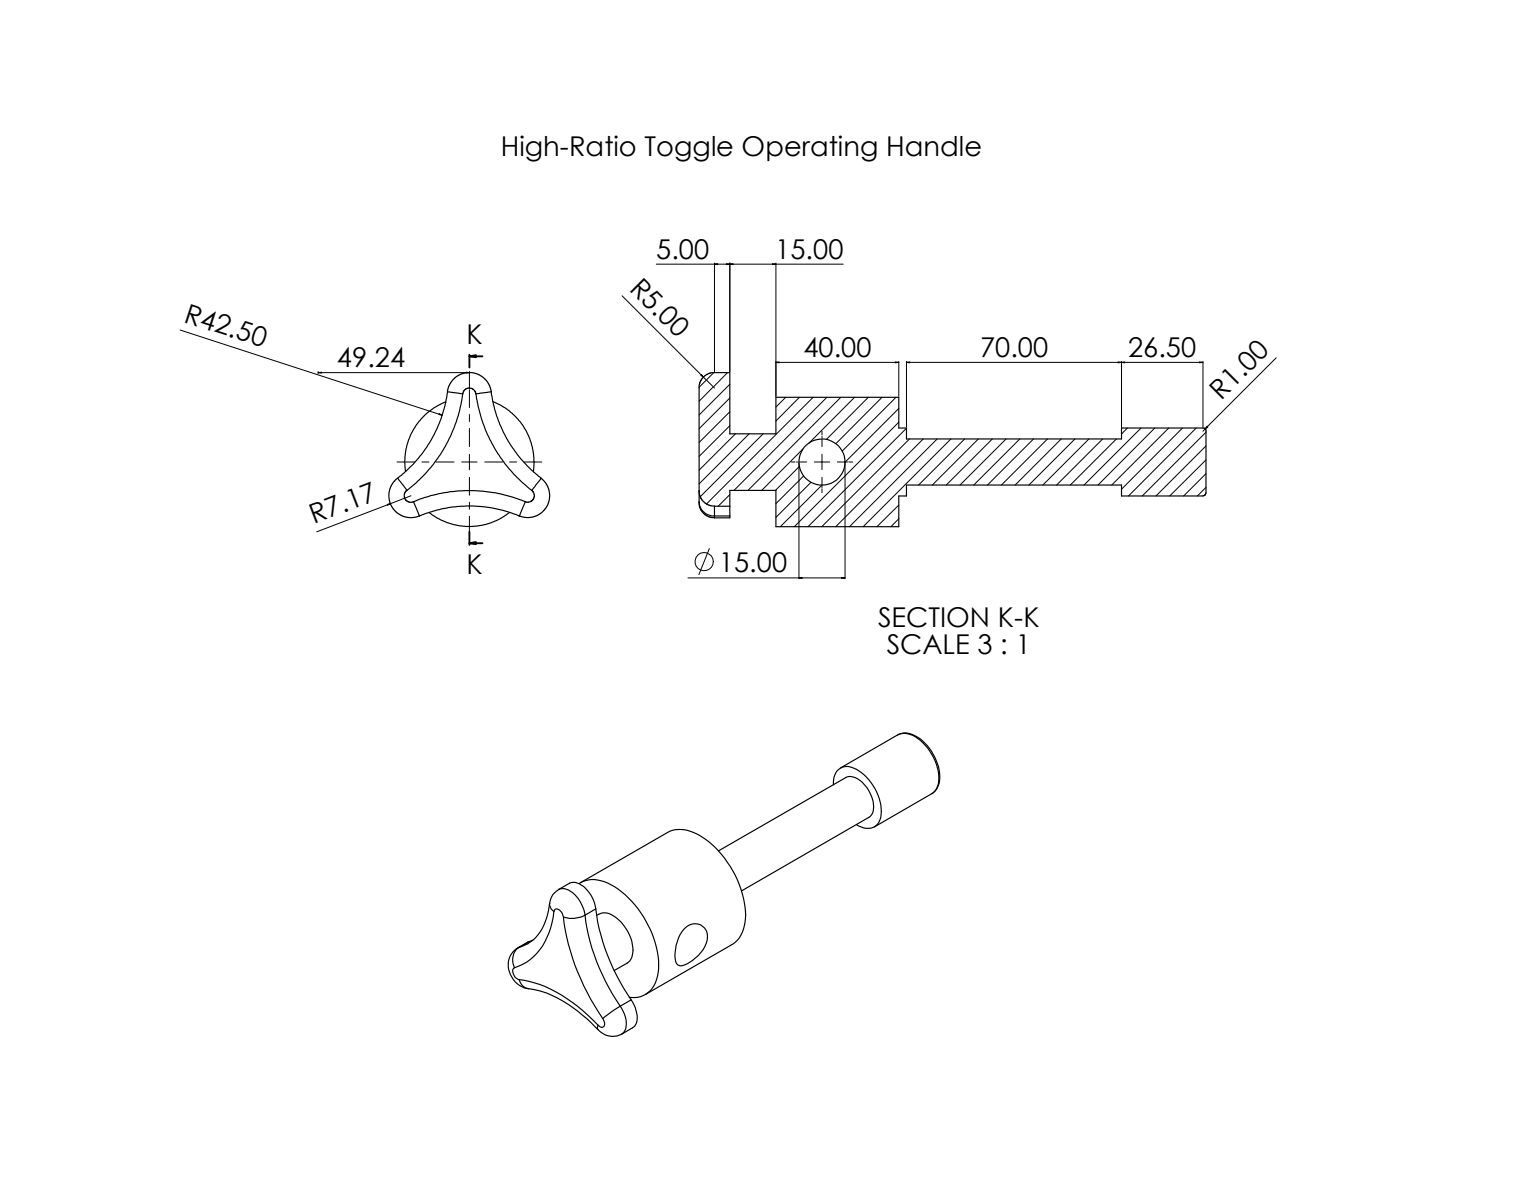
ISO-10303-21;
HEADER;
FILE_DESCRIPTION (('STEP AP214'),
    '1' );
FILE_NAME ('High-Ratio Toggle Operating Handle.step',
    '2026-10-21T18:33:49',
    ( '' ),
    ( '' ),
    'SwSTEP 2.0',
    'SolidWorks 2025',
    '' );
FILE_SCHEMA (( 'AUTOMOTIVE_DESIGN' ));
ENDSEC;

DATA;
#32=DIRECTION ( 'NONE',  ( -0.000000000000000000, -0.000000000000000000, -1.000000000000000000 ) ) ;
#36=AXIS2_PLACEMENT_3D ( 'NONE', #1369, #138, #1266 ) ;
#44=AXIS2_PLACEMENT_3D ( 'NONE', #11629, #14534, #15759 ) ;
#99=CARTESIAN_POINT ( 'NONE',  ( -57.08002265617300708, 84.22855780814606419, 35.00000000000000000 ) ) ;
#125=AXIS2_PLACEMENT_3D ( 'NONE', #2638, #18365, #4052 ) ;
#130=CYLINDRICAL_SURFACE ( 'NONE', #6082, 21.04359719766050318 ) ;
#138=DIRECTION ( 'NONE',  ( -0.000000000000000000, -0.000000000000000000, -1.000000000000000000 ) ) ;
#148=ORIENTED_EDGE ( 'NONE', *, *, #2746, .F. ) ;
#155=AXIS2_PLACEMENT_3D ( 'NONE', #551, #8645, #16166 ) ;
#219=ORIENTED_EDGE ( 'NONE', *, *, #12477, .T. ) ;
#259=CARTESIAN_POINT ( 'NONE',  ( -49.58002265617300708, 84.22855780814606419, 35.00000000000000000 ) ) ;
#264=CYLINDRICAL_SURFACE ( 'NONE', #16430, 21.04359719766050318 ) ;
#267=CARTESIAN_POINT ( 'NONE',  ( -38.92363814577095837, 71.26406042838981136, 102.5000000000000000 ) ) ;
#313=ORIENTED_EDGE ( 'NONE', *, *, #10756, .F. ) ;
#314=MANIFOLD_SOLID_BREP ( 'Cut-Extrude8', #12995 ) ;
#315=VERTEX_POINT ( 'NONE', #4152 ) ;
#323=DIRECTION ( 'NONE',  ( 0.000000000000000000, 0.000000000000000000, -1.000000000000000000 ) ) ;
#335=EDGE_CURVE ( 'NONE', #5779, #10128, #2839, .T. ) ;
#350=CARTESIAN_POINT ( 'NONE',  ( -83.23321842955245131, 73.26749283226919829, 97.49999999999998579 ) ) ;
#356=LINE ( 'NONE', #17469, #14795 ) ;
#358=CARTESIAN_POINT ( 'NONE',  ( -37.24050225201523290, 91.24541864506342392, 59.84040329251897816 ) ) ;
#361=ADVANCED_FACE ( 'NONE', ( #3024 ), #9005, .T. ) ;
#365=VECTOR ( 'NONE', #12626, 1000.000000000000000 ) ;
#377=CARTESIAN_POINT ( 'NONE',  ( -77.86181869377003295, 80.88798785482902076, 69.23289521281527925 ) ) ;
#408=LINE ( 'NONE', #4696, #15529 ) ;
#421=DIRECTION ( 'NONE',  ( -1.000000000000000000, 0.000000000000000000, 0.000000000000000000 ) ) ;
#449=CIRCLE ( 'NONE', #2236, 21.04359719766049608 ) ;
#456=DIRECTION ( 'NONE',  ( 0.000000000000000000, 0.000000000000000000, 1.000000000000000000 ) ) ;
#461=CARTESIAN_POINT ( 'NONE',  ( -36.29822661857599542, 80.88798785482900655, 55.76710478718474917 ) ) ;
#470=CARTESIAN_POINT ( 'NONE',  ( -73.32517902883354566, 66.64375664990241432, 102.5000000000000000 ) ) ;
#512=DIRECTION ( 'NONE',  ( 0.000000000000000000, 0.000000000000000000, 1.000000000000000000 ) ) ;
#534=CARTESIAN_POINT ( 'NONE',  ( -36.04074381574865527, 84.72093613475881568, 69.98790959730909833 ) ) ;
#551=CARTESIAN_POINT ( 'NONE',  ( -57.08002265617301418, 106.1506877598988154, 97.49999999999998579 ) ) ;
#554=ORIENTED_EDGE ( 'NONE', *, *, #15682, .F. ) ;
#569=TOROIDAL_SURFACE ( 'NONE', #11925, 10.04359719766049963, 1.000000000000000000 ) ;
#592=CIRCLE ( 'NONE', #14907, 7.168074330098680669 ) ;
#595=CARTESIAN_POINT ( 'NONE',  ( -78.12361985383350316, 84.22855780814606419, 77.50000000000000000 ) ) ;
#598=DIRECTION ( 'NONE',  ( 0.000000000000000000, 0.000000000000000000, 1.000000000000000000 ) ) ;
#604=AXIS2_PLACEMENT_3D ( 'NONE', #7949, #3633, #837 ) ;
#610=B_SPLINE_CURVE_WITH_KNOTS ( 'NONE', 3,
 ( #15647, #8545, #1426, #14249, #5805, #17565, #12326, #377, #10719, #3183, #10817, #4747, #15119, #3714, #16415, #3604, #897, #9324, #15203, #10926, #9506, #8984, #5202, #15020, #6601, #11795, #10297, #18019, #2389, #3804, #8096, #8894, #16611, #14677, #12219, #2299, #13815, #1004, #2211, #8002, #12429, #6705, #16072, #13198, #6066, #16515 ),
 .UNSPECIFIED., .F., .F.,
 ( 4, 2, 2, 2, 2, 2, 2, 2, 2, 2, 2, 2, 2, 2, 2, 2, 2, 2, 2, 2, 2, 2, 4 ),
 ( 1.387778780781445676E-17, 0.001477780233738794748, 0.002216670350608189195, 0.002955560467477583424, 0.004433340701216313337, 0.005172230818085679811, 0.005911120934955047153, 0.007388901168693846888, 0.008866681402432645756, 0.009605571519302056466, 0.01034446163617146891, 0.01182224186991029206, 0.01330002210364911869, 0.01477780233738794531, 0.01625558257112677193, 0.01699447268799620173, 0.01773336280486562805, 0.01921114303860447722, 0.01995003315547392089, 0.02068892327234336456, 0.02216670350608221027, 0.02290559362295161577, 0.02364448373982101781 ),
 .UNSPECIFIED. ) ;
#627=CIRCLE ( 'NONE', #12604, 47.49926016644946714 ) ;
#634=AXIS2_PLACEMENT_3D ( 'NONE', #7986, #512, #13420 ) ;
#641=EDGE_LOOP ( 'NONE', ( #13099, #15798 ) ) ;
#647=AXIS2_PLACEMENT_3D ( 'NONE', #8443, #1344, #3846 ) ;
#674=CARTESIAN_POINT ( 'NONE',  ( -76.06514409945376087, 73.26749283226919829, 97.49999999999998579 ) ) ;
#715=VERTEX_POINT ( 'NONE', #12761 ) ;
#718=DIRECTION ( 'NONE',  ( -1.000000000000000000, 0.000000000000000000, 0.000000000000000000 ) ) ;
#742=CARTESIAN_POINT ( 'NONE',  ( -36.67168494155210112, 79.09395985567564935, 57.02782509738743499 ) ) ;
#779=CARTESIAN_POINT ( 'NONE',  ( -76.88569266382195622, 91.34252568597634081, 60.07430202819471532 ) ) ;
#803=EDGE_CURVE ( 'NONE', #10920, #7762, #4578, .T. ) ;
#837=DIRECTION ( 'NONE',  ( 1.000000000000000000, 0.000000000000000000, 0.000000000000000000 ) ) ;
#851=UNCERTAINTY_MEASURE_WITH_UNIT (LENGTH_MEASURE( 1.000000000000000082E-05 ), #7064, 'distance_accuracy_value', 'NONE');
#856=CARTESIAN_POINT ( 'NONE',  ( -68.12361985383350316, 84.22855780814606419, 68.73600986863397111 ) ) ;
#861=CARTESIAN_POINT ( 'NONE',  ( -78.11930149659737310, 84.72093613475881568, 55.01209040269093720 ) ) ;
#868=FACE_OUTER_BOUND ( 'NONE', #12414, .T. ) ;
#872=EDGE_LOOP ( 'NONE', ( #7610, #14353 ) ) ;
#874=CARTESIAN_POINT ( 'NONE',  ( -38.92363814577095837, 71.26406042838981136, 97.49999999999998579 ) ) ;
#896=DIRECTION ( 'NONE',  ( -1.000000000000000000, 0.000000000000000000, 0.000000000000000000 ) ) ;
#897=CARTESIAN_POINT ( 'NONE',  ( -77.01756027604902499, 77.49305091727374872, 65.83480828159299847 ) ) ;
#918=ADVANCED_FACE ( 'NONE', ( #16269 ), #6147, .T. ) ;
#964=CARTESIAN_POINT ( 'NONE',  ( -77.95646096175848072, 86.88560906486408442, 69.51788182020753482 ) ) ;
#970=ORIENTED_EDGE ( 'NONE', *, *, #15172, .F. ) ;
#981=ORIENTED_EDGE ( 'NONE', *, *, #2192, .T. ) ;
#1004=CARTESIAN_POINT ( 'NONE',  ( -77.85981289659012816, 80.89962780276930232, 55.77475785633962602 ) ) ;
#1052=EDGE_CURVE ( 'NONE', #6388, #2078, #4951, .T. ) ;
#1066=ORIENTED_EDGE ( 'NONE', *, *, #5722, .T. ) ;
#1070=CARTESIAN_POINT ( 'NONE',  ( -77.35494310313409017, 89.87539756129700663, 67.45979609325928550 ) ) ;
#1071=EDGE_LOOP ( 'NONE', ( #14079, #1438 ) ) ;
#1095=ORIENTED_EDGE ( 'NONE', *, *, #8907, .T. ) ;
#1097=CYLINDRICAL_SURFACE ( 'NONE', #4269, 7.168074330098680669 ) ;
#1137=ORIENTED_EDGE ( 'NONE', *, *, #12714, .F. ) ;
#1180=DIRECTION ( 'NONE',  ( -1.000000000000000000, 0.000000000000000000, 0.000000000000000000 ) ) ;
#1186=ADVANCED_FACE ( 'NONE', ( #7022 ), #9528, .F. ) ;
#1207=CARTESIAN_POINT ( 'NONE',  ( -68.12361985383350316, 84.22855780814606419, 37.50000000000000000 ) ) ;
#1224=AXIS2_PLACEMENT_3D ( 'NONE', #99, #12928, #17214 ) ;
#1228=LINE ( 'NONE', #4398, #12878 ) ;
#1238=DIRECTION ( 'NONE',  ( 0.000000000000000000, 0.000000000000000000, 1.000000000000000000 ) ) ;
#1241=CARTESIAN_POINT ( 'NONE',  ( -83.23321842955245131, 73.26749283226919829, 92.50000000000000000 ) ) ;
#1252=CARTESIAN_POINT ( 'NONE',  ( -38.09490121289055509, 73.26749283227019305, 97.49999999999998579 ) ) ;
#1266=DIRECTION ( 'NONE',  ( -1.000000000000000000, 0.000000000000000000, 0.000000000000000000 ) ) ;
#1341=DIRECTION ( 'NONE',  ( -1.000000000000000000, 0.000000000000000000, 0.000000000000000000 ) ) ;
#1344=DIRECTION ( 'NONE',  ( -0.000000000000000000, 0.000000000000000000, -1.000000000000000000 ) ) ;
#1354=CARTESIAN_POINT ( 'NONE',  ( -76.06514409945376087, 73.26749283226919829, 102.5000000000000000 ) ) ;
#1355=VECTOR ( 'NONE', #4745, 1000.000000000000000 ) ;
#1369=CARTESIAN_POINT ( 'NONE',  ( -106.3193689061042164, 112.6569076202650450, 97.49999999999998579 ) ) ;
#1380=ORIENTED_EDGE ( 'NONE', *, *, #3456, .T. ) ;
#1395=DIRECTION ( 'NONE',  ( -0.000000000000000000, -0.000000000000000000, -1.000000000000000000 ) ) ;
#1420=EDGE_LOOP ( 'NONE', ( #3178, #16210, #16979, #14921 ) ) ;
#1426=CARTESIAN_POINT ( 'NONE',  ( -78.10583824988592028, 83.23774243329727085, 69.95051152545947559 ) ) ;
#1438=ORIENTED_EDGE ( 'NONE', *, *, #14205, .T. ) ;
#1441=CARTESIAN_POINT ( 'NONE',  ( -57.08002265617300708, 84.22855780814606419, 77.50000000000000000 ) ) ;
#1495=CARTESIAN_POINT ( 'NONE',  ( -57.08002265617300708, 84.22855780814606419, 92.50000000000000000 ) ) ;
#1508=CARTESIAN_POINT ( 'NONE',  ( -80.43148536604020649, 78.95224028009165806, 102.5000000000000000 ) ) ;
#1537=ORIENTED_EDGE ( 'NONE', *, *, #14930, .T. ) ;
#1540=DIRECTION ( 'NONE',  ( -1.000000000000000000, 0.000000000000000000, 0.000000000000000000 ) ) ;
#1583=CARTESIAN_POINT ( 'NONE',  ( -36.05803997522690452, 85.21341043856776309, 69.93917279341883386 ) ) ;
#1589=CYLINDRICAL_SURFACE ( 'NONE', #16728, 7.168074330099291736 ) ;
#1663=FACE_OUTER_BOUND ( 'NONE', #16501, .T. ) ;
#1672=DIRECTION ( 'NONE',  ( -1.000000000000000000, 0.000000000000000000, 0.000000000000000000 ) ) ;
#1676=CARTESIAN_POINT ( 'NONE',  ( -37.41836177203395408, 91.72869609463791107, 62.99211610237011172 ) ) ;
#1689=EDGE_CURVE ( 'NONE', #11390, #9243, #16057, .T. ) ;
#1711=PLANE ( 'NONE',  #44 ) ;
#1729=CARTESIAN_POINT ( 'NONE',  ( -76.06514409945376087, 73.26749283226919829, 92.50000000000000000 ) ) ;
#1735=CYLINDRICAL_SURFACE ( 'NONE', #9620, 9.197489084949710403 ) ;
#1758=CARTESIAN_POINT ( 'NONE',  ( -36.37230694946377696, 87.99602245404176415, 55.99668402450813431 ) ) ;
#1788=ORIENTED_EDGE ( 'NONE', *, *, #335, .F. ) ;
#1796=DIRECTION ( 'NONE',  ( 0.3822456275482439270, -0.9240607556975077852, 0.000000000000000000 ) ) ;
#1801=LINE ( 'NONE', #8920, #18007 ) ;
#1853=DIRECTION ( 'NONE',  ( -0.000000000000000000, -0.000000000000000000, -1.000000000000000000 ) ) ;
#1862=CARTESIAN_POINT ( 'NONE',  ( -36.12589806422543148, 82.27553650601718971, 55.25452123045118213 ) ) ;
#1872=CIRCLE ( 'NONE', #13239, 9.197489084949710403 ) ;
#1953=DIRECTION ( 'NONE',  ( 1.000000000000000000, 0.000000000000000000, -0.000000000000000000 ) ) ;
#1970=DIRECTION ( 'NONE',  ( 1.000000000000000000, 0.000000000000000000, 0.000000000000000000 ) ) ;
#1978=B_SPLINE_CURVE_WITH_KNOTS ( 'NONE', 3,
 ( #4661, #10374, #3254, #14669, #1862, #7570, #13280, #461, #10834, #4010, #15036, #9438, #742, #17932, #9522, #17844, #6619, #11027, #6520, #2229, #3622, #15132, #2314, #16531, #9723, #7941, #8020, #6435, #5117, #15224, #5021, #12343, #16712, #12236, #9616, #2410, #2612, #10940, #13733, #15320, #12533, #13651, #8116, #6724, #13554, #6812 ),
 .UNSPECIFIED., .F., .F.,
 ( 4, 2, 2, 2, 2, 2, 2, 2, 2, 2, 2, 2, 2, 2, 2, 2, 2, 2, 2, 2, 2, 2, 4 ),
 ( 0.000000000000000000, 0.001477780233738735334, 0.002216670350608105061, 0.002955560467477474570, 0.004433340701216251754, 0.005172230818085658995, 0.005911120934955066235, 0.007388901168693925818, 0.008866681402432782799, 0.009605571519302205652, 0.01034446163617162677, 0.01182224186991048982, 0.01330002210364935461, 0.01477780233738821593, 0.01625558257112707725, 0.01699447268799647928, 0.01773336280486588479, 0.01921114303860466457, 0.01995003315547405273, 0.02068892327234343395, 0.02216670350608219292, 0.02290559362295159149, 0.02364448373982099005 ),
 .UNSPECIFIED. ) ;
#1991=CARTESIAN_POINT ( 'NONE',  ( -76.83309350041878361, 91.48526692943183036, 60.54251226750088222 ) ) ;
#1994=DIRECTION ( 'NONE',  ( -1.000000000000000000, 0.000000000000000000, 0.000000000000000000 ) ) ;
#2010=EDGE_CURVE ( 'NONE', #8653, #11390, #6438, .T. ) ;
#2014=ORIENTED_EDGE ( 'NONE', *, *, #2838, .F. ) ;
#2026=CARTESIAN_POINT ( 'NONE',  ( -47.88253357122329845, 84.22855780814606419, 92.50000000000000000 ) ) ;
#2064=EDGE_CURVE ( 'NONE', #14012, #2549, #12075, .T. ) ;
#2078=VERTEX_POINT ( 'NONE', #3533 ) ;
#2092=ORIENTED_EDGE ( 'NONE', *, *, #4008, .T. ) ;
#2169=CARTESIAN_POINT ( 'NONE',  ( -78.23321842955243710, 73.26749283226919829, 97.49999999999998579 ) ) ;
#2173=FACE_OUTER_BOUND ( 'NONE', #18405, .T. ) ;
#2181=AXIS2_PLACEMENT_3D ( 'NONE', #6034, #4384, #2976 ) ;
#2192=EDGE_CURVE ( 'NONE', #8653, #10149, #14444, .T. ) ;
#2194=( GEOMETRIC_REPRESENTATION_CONTEXT ( 3 ) GLOBAL_UNCERTAINTY_ASSIGNED_CONTEXT ( ( #12468 ) ) GLOBAL_UNIT_ASSIGNED_CONTEXT ( ( #10446, #10543, #16139 ) ) REPRESENTATION_CONTEXT ( 'NONE', 'WORKASPACE' ) );
#2195=AXIS2_PLACEMENT_3D ( 'NONE', #3510, #5002, #17909 ) ;
#2211=CARTESIAN_POINT ( 'NONE',  ( -77.89415131665849401, 81.12099773066752562, 55.66971324650689468 ) ) ;
#2227=PRODUCT_DEFINITION ( 'UNKNOWN', '', #11173, #6257 ) ;
#2229=CARTESIAN_POINT ( 'NONE',  ( -37.32251811057857793, 76.98425793134822470, 60.54272255928178481 ) ) ;
#2236=AXIS2_PLACEMENT_3D ( 'NONE', #5521, #18049, #2427 ) ;
#2248=EDGE_CURVE ( 'NONE', #4300, #12168, #2317, .T. ) ;
#2259=DIRECTION ( 'NONE',  ( -0.000000000000000000, -0.000000000000000000, -1.000000000000000000 ) ) ;
#2299=CARTESIAN_POINT ( 'NONE',  ( -77.74594894602464024, 80.25424057604627137, 56.13491590375404172 ) ) ;
#2314=CARTESIAN_POINT ( 'NONE',  ( -37.41820911104731806, 76.72881973191589111, 62.00219528655608059 ) ) ;
#2317=LINE ( 'NONE', #8024, #6348 ) ;
#2340=DIRECTION ( 'NONE',  ( -0.000000000000000000, -0.000000000000000000, -1.000000000000000000 ) ) ;
#2343=CARTESIAN_POINT ( 'NONE',  ( -40.83486628351231218, 66.64375664990294013, 97.49999999999998579 ) ) ;
#2389=CARTESIAN_POINT ( 'NONE',  ( -77.09623126797262671, 77.72742355542474968, 58.72881290435446289 ) ) ;
#2400=ADVANCED_FACE ( 'NONE', ( #1663 ), #16049, .T. ) ;
#2408=CARTESIAN_POINT ( 'NONE',  ( -57.08002265617300708, 84.22855780814606419, 68.73600986863397111 ) ) ;
#2410=CARTESIAN_POINT ( 'NONE',  ( -36.41409636632135971, 80.25424057604624295, 68.86508409624599381 ) ) ;
#2414=EDGE_CURVE ( 'NONE', #10920, #17012, #10253, .T. ) ;
#2421=EDGE_CURVE ( 'NONE', #17891, #4300, #13836, .T. ) ;
#2427=DIRECTION ( 'NONE',  ( 1.000000000000000000, 0.000000000000000000, 0.000000000000000000 ) ) ;
#2453=CARTESIAN_POINT ( 'NONE',  ( -76.76049879875490944, 91.67990741037235125, 63.48630363751230021 ) ) ;
#2462=AXIS2_PLACEMENT_3D ( 'NONE', #6172, #2259, #13314 ) ;
#2467=DIRECTION ( 'NONE',  ( -0.000000000000000000, -0.000000000000000000, 1.000000000000000000 ) ) ;
#2484=CARTESIAN_POINT ( 'NONE',  ( -7.840676406241780860, 112.6569076202650308, 92.50000000000000000 ) ) ;
#2499=ORIENTED_EDGE ( 'NONE', *, *, #12714, .T. ) ;
#2514=ORIENTED_EDGE ( 'NONE', *, *, #3214, .T. ) ;
#2549=VERTEX_POINT ( 'NONE', #16234 ) ;
#2563=CARTESIAN_POINT ( 'NONE',  ( -78.12361985383350316, 84.22855780814607840, 70.00000000000001421 ) ) ;
#2586=CARTESIAN_POINT ( 'NONE',  ( -57.08002265617300708, 84.22855780814606419, 35.00000000000000000 ) ) ;
#2589=CARTESIAN_POINT ( 'NONE',  ( -54.93063083320800644, 106.4346967249107792, 97.49999999999998579 ) ) ;
#2594=DIRECTION ( 'NONE',  ( -1.224646799147353207E-16, 1.000000000000000000, 0.000000000000000000 ) ) ;
#2597=DIRECTION ( 'NONE',  ( -0.000000000000000000, -0.000000000000000000, -1.000000000000000000 ) ) ;
#2612=CARTESIAN_POINT ( 'NONE',  ( -36.37443156682203949, 80.46558623543624833, 68.99235718476280965 ) ) ;
#2622=DIRECTION ( 'NONE',  ( -1.000000000000000000, 0.000000000000000000, 0.000000000000000000 ) ) ;
#2627=ORIENTED_EDGE ( 'NONE', *, *, #12477, .F. ) ;
#2638=CARTESIAN_POINT ( 'NONE',  ( -38.09490121289055509, 73.26749283227019305, 97.49999999999998579 ) ) ;
#2653=FACE_OUTER_BOUND ( 'NONE', #13653, .T. ) ;
#2657=EDGE_CURVE ( 'NONE', #17012, #4505, #3991, .T. ) ;
#2670=ORIENTED_EDGE ( 'NONE', *, *, #14218, .T. ) ;
#2671=PLANE ( 'NONE',  #15226 ) ;
#2687=CARTESIAN_POINT ( 'NONE',  ( -57.08002265617300708, 84.22855780814606419, -35.00000000000000000 ) ) ;
#2693=LINE ( 'NONE', #6714, #365 ) ;
#2746=EDGE_CURVE ( 'NONE', #5564, #15197, #8172, .T. ) ;
#2747=EDGE_LOOP ( 'NONE', ( #8359, #11367 ) ) ;
#2749=DIRECTION ( 'NONE',  ( 0.000000000000000000, 0.000000000000000000, -1.000000000000000000 ) ) ;
#2778=EDGE_CURVE ( 'NONE', #15227, #15032, #7428, .T. ) ;
#2786=VERTEX_POINT ( 'NONE', #595 ) ;
#2838=EDGE_CURVE ( 'NONE', #9739, #15151, #17147, .T. ) ;
#2839=CIRCLE ( 'NONE', #13284, 10.04359719766049430 ) ;
#2890=DIRECTION ( 'NONE',  ( -1.000000000000000000, 0.000000000000000000, 0.000000000000000000 ) ) ;
#2893=ADVANCED_FACE ( 'NONE', ( #5274 ), #16765, .T. ) ;
#2911=EDGE_CURVE ( 'NONE', #15151, #8454, #17991, .T. ) ;
#2935=FACE_OUTER_BOUND ( 'NONE', #17821, .T. ) ;
#2938=ADVANCED_FACE ( 'NONE', ( #2935 ), #130, .T. ) ;
#2944=DIRECTION ( 'NONE',  ( -1.000000000000000000, 0.000000000000000000, 0.000000000000000000 ) ) ;
#2963=CARTESIAN_POINT ( 'NONE',  ( -64.18632899337946185, 107.0896764944433954, 102.5000000000000000 ) ) ;
#2976=DIRECTION ( 'NONE',  ( -1.000000000000000000, -1.632709340522812220E-15, 0.000000000000000000 ) ) ;
#2990=CARTESIAN_POINT ( 'NONE',  ( -37.13913369598539305, 90.95230598576922887, 65.83182832201505619 ) ) ;
#2991=DIRECTION ( 'NONE',  ( 1.000000000000000000, 0.000000000000000000, 0.000000000000000000 ) ) ;
#3013=ORIENTED_EDGE ( 'NONE', *, *, #17161, .T. ) ;
#3024=FACE_OUTER_BOUND ( 'NONE', #1420, .T. ) ;
#3030=FACE_OUTER_BOUND ( 'NONE', #3216, .T. ) ;
#3040=ORIENTED_EDGE ( 'NONE', *, *, #15682, .T. ) ;
#3059=CARTESIAN_POINT ( 'NONE',  ( -78.12361985383350316, 84.22855780814606419, 37.50000000000000000 ) ) ;
#3077=CARTESIAN_POINT ( 'NONE',  ( -37.02218768164058815, 90.59536451873519525, 66.47148242010926822 ) ) ;
#3095=DIRECTION ( 'NONE',  ( -1.000000000000000000, 0.000000000000000000, 0.000000000000000000 ) ) ;
#3136=CARTESIAN_POINT ( 'NONE',  ( -57.08002265617300708, 84.22855780814606419, 37.50000000000000000 ) ) ;
#3155=CIRCLE ( 'NONE', #8835, 42.49926016644912607 ) ;
#3165=CARTESIAN_POINT ( 'NONE',  ( -66.27751174112272281, 84.22855780814606419, 77.50000000000000000 ) ) ;
#3172=CARTESIAN_POINT ( 'NONE',  ( -37.06251219239532446, 90.72064142110004070, 58.73664414705599768 ) ) ;
#3173=PLANE ( 'NONE',  #17051 ) ;
#3178=ORIENTED_EDGE ( 'NONE', *, *, #4773, .F. ) ;
#3183=CARTESIAN_POINT ( 'NONE',  ( -77.66397652102858729, 79.84943054288078201, 68.59368636907963435 ) ) ;
#3194=DIRECTION ( 'NONE',  ( 1.000000000000000000, 0.000000000000000000, 0.000000000000000000 ) ) ;
#3214=EDGE_CURVE ( 'NONE', #15197, #15151, #12698, .T. ) ;
#3216=EDGE_LOOP ( 'NONE', ( #8491, #17094, #10489, #14441 ) ) ;
#3239=DIRECTION ( 'NONE',  ( -1.000000000000000000, 0.000000000000000000, -0.000000000000000000 ) ) ;
#3243=AXIS2_PLACEMENT_3D ( 'NONE', #10958, #9363, #16732 ) ;
#3254=CARTESIAN_POINT ( 'NONE',  ( -36.05420706246012230, 83.23774243329727085, 55.04948847454055283 ) ) ;
#3281=CIRCLE ( 'NONE', #7774, 7.168074330098680669 ) ;
#3310=EDGE_CURVE ( 'NONE', #15460, #7762, #15952, .T. ) ;
#3336=CARTESIAN_POINT ( 'NONE',  ( -83.23321842955245131, 73.26749283226919829, 102.5000000000000000 ) ) ;
#3339=CARTESIAN_POINT ( 'NONE',  ( -36.29790135706344500, 87.56725157785861313, 55.76609545620163999 ) ) ;
#3366=EDGE_LOOP ( 'NONE', ( #8412, #7266 ) ) ;
#3373=AXIS2_PLACEMENT_3D ( 'NONE', #5947, #13260, #14388 ) ;
#3383=CARTESIAN_POINT ( 'NONE',  ( -77.02091161636059269, 90.95230598576924308, 59.16817167798495802 ) ) ;
#3410=EDGE_CURVE ( 'NONE', #15435, #4264, #6845, .T. ) ;
#3431=AXIS2_PLACEMENT_3D ( 'NONE', #2589, #9692, #6880 ) ;
#3448=EDGE_LOOP ( 'NONE', ( #17964, #7792, #4837, #16368, #8677, #11944, #5495 ) ) ;
#3456=EDGE_CURVE ( 'NONE', #2549, #14012, #610, .T. ) ;
#3463=DIRECTION ( 'NONE',  ( 0.000000000000000000, 0.000000000000000000, 1.000000000000000000 ) ) ;
#3480=DIRECTION ( 'NONE',  ( 0.000000000000000000, 0.000000000000000000, -1.000000000000000000 ) ) ;
#3497=CARTESIAN_POINT ( 'NONE',  ( -36.03642545851251100, 84.22855780814606419, 37.50000000000000000 ) ) ;
#3505=DIRECTION ( 'NONE',  ( -1.000000000000000000, 0.000000000000000000, 0.000000000000000000 ) ) ;
#3510=CARTESIAN_POINT ( 'NONE',  ( -57.08002265617300708, 84.22855780814606419, 77.50000000000000000 ) ) ;
#3533=CARTESIAN_POINT ( 'NONE',  ( -73.32517902883354566, 66.64375664990241432, 92.50000000000000000 ) ) ;
#3563=DIRECTION ( 'NONE',  ( -0.000000000000000000, -0.000000000000000000, -1.000000000000000000 ) ) ;
#3564=AXIS2_PLACEMENT_3D ( 'NONE', #674, #3563, #6757 ) ;
#3569=CARTESIAN_POINT ( 'NONE',  ( -77.62243764337172536, 88.81248391902214223, 56.54393065445481881 ) ) ;
#3571=ORIENTED_EDGE ( 'NONE', *, *, #4773, .T. ) ;
#3572=FACE_OUTER_BOUND ( 'NONE', #9361, .T. ) ;
#3577=AXIS2_PLACEMENT_3D ( 'NONE', #13659, #12355, #4954 ) ;
#3604=CARTESIAN_POINT ( 'NONE',  ( -77.09486422618832080, 77.72307496574235586, 66.26442681581322347 ) ) ;
#3614=ORIENTED_EDGE ( 'NONE', *, *, #14205, .F. ) ;
#3622=CARTESIAN_POINT ( 'NONE',  ( -37.34515446474368616, 76.92303621577349304, 60.78520344204553538 ) ) ;
#3623=ORIENTED_EDGE ( 'NONE', *, *, #2064, .F. ) ;
#3633=DIRECTION ( 'NONE',  ( -0.000000000000000000, -0.000000000000000000, -1.000000000000000000 ) ) ;
#3677=FACE_OUTER_BOUND ( 'NONE', #6379, .T. ) ;
#3682=AXIS2_PLACEMENT_3D ( 'NONE', #17936, #9442, #16535 ) ;
#3712=CARTESIAN_POINT ( 'NONE',  ( -36.03642545851251100, 84.22855780814606419, 77.50000000000000000 ) ) ;
#3714=CARTESIAN_POINT ( 'NONE',  ( -77.35440395286859427, 78.57985073358727846, 67.45754834358830010 ) ) ;
#3724=AXIS2_PLACEMENT_3D ( 'NONE', #2687, #9894, #8499 ) ;
#3735=AXIS2_PLACEMENT_3D ( 'NONE', #13528, #5193, #3505 ) ;
#3746=ORIENTED_EDGE ( 'NONE', *, *, #2192, .F. ) ;
#3750=DIRECTION ( 'NONE',  ( -0.000000000000000000, -0.000000000000000000, -1.000000000000000000 ) ) ;
#3752=ORIENTED_EDGE ( 'NONE', *, *, #8089, .F. ) ;
#3759=ADVANCED_FACE ( 'NONE', ( #10246 ), #14466, .T. ) ;
#3760=LINE ( 'NONE', #856, #8958 ) ;
#3765=VERTEX_POINT ( 'NONE', #14629 ) ;
#3780=EDGE_CURVE ( 'NONE', #4264, #10128, #7159, .T. ) ;
#3800=DIRECTION ( 'NONE',  ( -0.000000000000000000, -0.000000000000000000, -1.000000000000000000 ) ) ;
#3804=CARTESIAN_POINT ( 'NONE',  ( -77.22213323485729575, 78.13360439242252653, 58.12270716872546927 ) ) ;
#3819=ORIENTED_EDGE ( 'NONE', *, *, #14218, .F. ) ;
#3846=DIRECTION ( 'NONE',  ( -1.000000000000000000, 0.000000000000000000, 0.000000000000000000 ) ) ;
#3883=ORIENTED_EDGE ( 'NONE', *, *, #5854, .F. ) ;
#3885=CARTESIAN_POINT ( 'NONE',  ( -35.92682688279126779, 73.26749283227019305, 97.49999999999998579 ) ) ;
#3893=ADVANCED_FACE ( 'NONE', ( #18398, #15289 ), #2671, .F. ) ;
#3915=AXIS2_PLACEMENT_3D ( 'NONE', #14702, #7413, #1796 ) ;
#3921=AXIS2_PLACEMENT_3D ( 'NONE', #16023, #10138, #2944 ) ;
#3924=ORIENTED_EDGE ( 'NONE', *, *, #16449, .T. ) ;
#3943=FACE_OUTER_BOUND ( 'NONE', #3448, .T. ) ;
#3946=DIRECTION ( 'NONE',  ( 1.000000000000000000, 0.000000000000000000, 0.000000000000000000 ) ) ;
#3948=CARTESIAN_POINT ( 'NONE',  ( -77.53399986885767703, 89.18779308299872355, 68.14733228818110433 ) ) ;
#3957=ORIENTED_EDGE ( 'NONE', *, *, #4008, .F. ) ;
#3959=AXIS2_PLACEMENT_3D ( 'NONE', #14352, #7416, #1540 ) ;
#3973=CARTESIAN_POINT ( 'NONE',  ( -38.09490121289055509, 73.26749283227019305, 102.5000000000000000 ) ) ;
#3980=ORIENTED_EDGE ( 'NONE', *, *, #5034, .T. ) ;
#3991=CIRCLE ( 'NONE', #10264, 4.999999999999998224 ) ;
#4008=EDGE_CURVE ( 'NONE', #8703, #8868, #4519, .T. ) ;
#4010=CARTESIAN_POINT ( 'NONE',  ( -36.49606879131744108, 79.84943054288081044, 56.40631363092040829 ) ) ;
#4011=ORIENTED_EDGE ( 'NONE', *, *, #2838, .T. ) ;
#4036=ORIENTED_EDGE ( 'NONE', *, *, #1052, .T. ) ;
#4038=EDGE_CURVE ( 'NONE', #715, #6290, #9548, .T. ) ;
#4045=AXIS2_PLACEMENT_3D ( 'NONE', #5357, #8370, #11465 ) ;
#4052=DIRECTION ( 'NONE',  ( -1.000000000000000000, 0.000000000000000000, 0.000000000000000000 ) ) ;
#4082=CARTESIAN_POINT ( 'NONE',  ( -76.06514409945376087, 73.26749283226919829, 102.5000000000000000 ) ) ;
#4089=ORIENTED_EDGE ( 'NONE', *, *, #4353, .T. ) ;
#4130=ADVANCED_FACE ( 'NONE', ( #2173 ), #569, .T. ) ;
#4147=VERTEX_POINT ( 'NONE', #10690 ) ;
#4148=DIRECTION ( 'NONE',  ( -1.000000000000000000, 0.000000000000000000, 0.000000000000000000 ) ) ;
#4150=ADVANCED_FACE ( 'NONE', ( #3572 ), #9113, .T. ) ;
#4152=CARTESIAN_POINT ( 'NONE',  ( -64.58002265617299997, 84.22855780814606419, -35.00000000000000000 ) ) ;
#4153=CIRCLE ( 'NONE', #6834, 11.04359719766050141 ) ;
#4167=ORIENTED_EDGE ( 'NONE', *, *, #2778, .F. ) ;
#4239=EDGE_CURVE ( 'NONE', #2549, #7660, #408, .T. ) ;
#4264=VERTEX_POINT ( 'NONE', #15167 ) ;
#4269=AXIS2_PLACEMENT_3D ( 'NONE', #4082, #12700, #18399 ) ;
#4292=CYLINDRICAL_SURFACE ( 'NONE', #15254, 42.49926016645017057 ) ;
#4299=CARTESIAN_POINT ( 'NONE',  ( -68.12361985383350316, 84.22855780814606419, -35.00000000000000000 ) ) ;
#4300=VERTEX_POINT ( 'NONE', #5167 ) ;
#4332=CYLINDRICAL_SURFACE ( 'NONE', #15784, 7.168074330098680669 ) ;
#4353=EDGE_CURVE ( 'NONE', #14012, #8703, #6952, .T. ) ;
#4356=TOROIDAL_SURFACE ( 'NONE', #10326, 2.168074330098679336, 5.000000000000000000 ) ;
#4384=DIRECTION ( 'NONE',  ( 0.000000000000000000, 0.000000000000000000, 1.000000000000000000 ) ) ;
#4398=CARTESIAN_POINT ( 'NONE',  ( -68.12361985383350316, 84.22855780814606419, 68.73600986863397111 ) ) ;
#4423=AXIS2_PLACEMENT_3D ( 'NONE', #11226, #6905, #12633 ) ;
#4426=CARTESIAN_POINT ( 'NONE',  ( -67.12361985383350316, 84.22855780814606419, -62.50000000000000000 ) ) ;
#4455=ORIENTED_EDGE ( 'NONE', *, *, #17733, .T. ) ;
#4472=CARTESIAN_POINT ( 'NONE',  ( -37.32695181192723766, 91.48526692943180194, 64.45748773249914620 ) ) ;
#4487=AXIS2_PLACEMENT_3D ( 'NONE', #13276, #456, #17555 ) ;
#4490=CARTESIAN_POINT ( 'NONE',  ( -38.09490121289055509, 73.26749283227019305, 92.50000000000000000 ) ) ;
#4491=AXIS2_PLACEMENT_3D ( 'NONE', #14233, #11140, #2622 ) ;
#4494=ORIENTED_EDGE ( 'NONE', *, *, #2421, .T. ) ;
#4505=VERTEX_POINT ( 'NONE', #16080 ) ;
#4510=EDGE_LOOP ( 'NONE', ( #10998, #14670, #13034, #13949 ) ) ;
#4519=LINE ( 'NONE', #10060, #6549 ) ;
#4545=TOROIDAL_SURFACE ( 'NONE', #2462, 2.168074330099288183, 5.000000000000000000 ) ;
#4560=CARTESIAN_POINT ( 'NONE',  ( -37.39954651359116866, 91.67990741037236546, 61.51369636248775663 ) ) ;
#4562=EDGE_CURVE ( 'NONE', #18509, #14448, #18232, .T. ) ;
#4578=LINE ( 'NONE', #1508, #17754 ) ;
#4584=AXIS2_PLACEMENT_3D ( 'NONE', #8855, #11835, #4704 ) ;
#4654=CARTESIAN_POINT ( 'NONE',  ( -57.08002265617302839, 27.37185818390810965, 97.49999999999998579 ) ) ;
#4656=CARTESIAN_POINT ( 'NONE',  ( -36.03642545851251100, 84.22855780814606419, 70.00000000000001421 ) ) ;
#4661=CARTESIAN_POINT ( 'NONE',  ( -36.03642545851251100, 84.22855780814606419, 55.00000000000001421 ) ) ;
#4696=CARTESIAN_POINT ( 'NONE',  ( -123.4618227840623632, 84.22855780814606419, 70.00000000000001421 ) ) ;
#4699=CARTESIAN_POINT ( 'NONE',  ( -123.4618227840623632, 84.22855780814606419, 62.50000000000001421 ) ) ;
#4703=DIRECTION ( 'NONE',  ( 0.9240607556974789194, -0.3822456275483139820, 0.000000000000000000 ) ) ;
#4704=DIRECTION ( 'NONE',  ( 0.000000000000000000, 0.000000000000000000, -1.000000000000000000 ) ) ;
#4720=EDGE_LOOP ( 'NONE', ( #2627, #14260 ) ) ;
#4725=DIRECTION ( 'NONE',  ( 0.000000000000000000, 0.000000000000000000, 1.000000000000000000 ) ) ;
#4733=CARTESIAN_POINT ( 'NONE',  ( -37.17548309439882104, 91.05880801963004956, 65.60778368822992945 ) ) ;
#4745=DIRECTION ( 'NONE',  ( -0.000000000000000000, -0.000000000000000000, -1.000000000000000000 ) ) ;
#4747=CARTESIAN_POINT ( 'NONE',  ( -77.53293207630810002, 79.27386099610181702, 68.13566487288508711 ) ) ;
#4773=EDGE_CURVE ( 'NONE', #16002, #4147, #14648, .T. ) ;
#4776=CARTESIAN_POINT ( 'NONE',  ( -77.26346150264693335, 90.19024662095813483, 57.92355293790617310 ) ) ;
#4794=CARTESIAN_POINT ( 'NONE',  ( -36.03642545851251100, 84.22855780814606419, 70.00000000000001421 ) ) ;
#4808=AXIS2_PLACEMENT_3D ( 'NONE', #9285, #9466, #3946 ) ;
#4824=CARTESIAN_POINT ( 'NONE',  ( -57.08002265617300708, 84.22855780814606419, 92.50000000000000000 ) ) ;
#4837=ORIENTED_EDGE ( 'NONE', *, *, #13828, .F. ) ;
#4867=AXIS2_PLACEMENT_3D ( 'NONE', #12891, #14204, #5579 ) ;
#4870=VECTOR ( 'NONE', #15384, 1000.000000000000000 ) ;
#4890=PRODUCT_DEFINITION_SHAPE ( 'NONE', 'NONE',  #2227 ) ;
#4928=ORIENTED_EDGE ( 'NONE', *, *, #15172, .T. ) ;
#4931=AXIS2_PLACEMENT_3D ( 'NONE', #4654, #10368, #9152 ) ;
#4939=DIRECTION ( 'NONE',  ( 0.000000000000000000, 0.000000000000000000, 1.000000000000000000 ) ) ;
#4944=DIRECTION ( 'NONE',  ( -1.000000000000000000, 0.000000000000000000, 0.000000000000000000 ) ) ;
#4951=LINE ( 'NONE', #470, #1355 ) ;
#4954=DIRECTION ( 'NONE',  ( -1.000000000000000000, 0.000000000000000000, 0.000000000000000000 ) ) ;
#4976=DIRECTION ( 'NONE',  ( 0.000000000000000000, 0.000000000000000000, -1.000000000000000000 ) ) ;
#4998=ADVANCED_FACE ( 'NONE', ( #17374, #10371 ), #3173, .T. ) ;
#5002=DIRECTION ( 'NONE',  ( 0.000000000000000000, 0.000000000000000000, 1.000000000000000000 ) ) ;
#5003=ORIENTED_EDGE ( 'NONE', *, *, #2657, .T. ) ;
#5021=CARTESIAN_POINT ( 'NONE',  ( -36.89438688693570612, 78.27883601870421160, 67.07281572422797922 ) ) ;
#5024=ORIENTED_EDGE ( 'NONE', *, *, #13214, .F. ) ;
#5034=EDGE_CURVE ( 'NONE', #9243, #2078, #5695, .T. ) ;
#5043=ORIENTED_EDGE ( 'NONE', *, *, #3310, .T. ) ;
#5062=CARTESIAN_POINT ( 'NONE',  ( -78.12361985383353158, 84.47473112397163675, 55.00000000000002132 ) ) ;
#5065=CARTESIAN_POINT ( 'NONE',  ( -123.4618227840623632, 84.22855780814606419, 55.00000000000001421 ) ) ;
#5117=CARTESIAN_POINT ( 'NONE',  ( -37.06381404437335902, 77.72742355542473547, 66.27118709564553001 ) ) ;
#5133=EDGE_CURVE ( 'NONE', #5248, #7744, #18254, .T. ) ;
#5167=CARTESIAN_POINT ( 'NONE',  ( -33.72855994630469212, 78.95224028009285178, 97.49999999999998579 ) ) ;
#5171=ORIENTED_EDGE ( 'NONE', *, *, #16689, .T. ) ;
#5193=DIRECTION ( 'NONE',  ( 0.000000000000000000, 0.000000000000000000, 1.000000000000000000 ) ) ;
#5202=CARTESIAN_POINT ( 'NONE',  ( -76.74183620129869610, 76.72881973191590532, 62.99780471344396204 ) ) ;
#5248=VERTEX_POINT ( 'NONE', #7098 ) ;
#5260=ORIENTED_EDGE ( 'NONE', *, *, #803, .F. ) ;
#5273=EDGE_CURVE ( 'NONE', #10920, #13449, #12197, .T. ) ;
#5274=FACE_OUTER_BOUND ( 'NONE', #12522, .T. ) ;
#5309=DIRECTION ( 'NONE',  ( 1.000000000000000000, 0.000000000000000000, 0.000000000000000000 ) ) ;
#5340=CARTESIAN_POINT ( 'NONE',  ( -64.18632899337946185, 107.0896764944433954, 97.49999999999998579 ) ) ;
#5341=CARTESIAN_POINT ( 'NONE',  ( -77.02089413874927004, 90.95236025322215312, 65.83173792382639533 ) ) ;
#5351=EDGE_CURVE ( 'NONE', #4300, #15197, #14004, .T. ) ;
#5357=CARTESIAN_POINT ( 'NONE',  ( -57.08002265617301418, 106.1506877598988154, 97.49999999999998579 ) ) ;
#5367=EDGE_LOOP ( 'NONE', ( #14926, #1137, #2014, #16275 ) ) ;
#5383=CIRCLE ( 'NONE', #4491, 11.04359719766049430 ) ;
#5396=ORIENTED_EDGE ( 'NONE', *, *, #3780, .F. ) ;
#5398=ADVANCED_FACE ( 'NONE', ( #3677 ), #17520, .F. ) ;
#5403=FACE_OUTER_BOUND ( 'NONE', #10010, .T. ) ;
#5421=EDGE_LOOP ( 'NONE', ( #313, #6789, #18169, #8117 ) ) ;
#5442=ORIENTED_EDGE ( 'NONE', *, *, #17161, .F. ) ;
#5481=ADVANCED_FACE ( 'NONE', ( #868 ), #14585, .T. ) ;
#5495=ORIENTED_EDGE ( 'NONE', *, *, #14997, .F. ) ;
#5502=CARTESIAN_POINT ( 'NONE',  ( -106.3193689061042164, 112.6569076202650450, 102.5000000000000000 ) ) ;
#5508=ADVANCED_FACE ( 'NONE', ( #2653 ), #5550, .F. ) ;
#5521=CARTESIAN_POINT ( 'NONE',  ( -57.08002265617300708, 84.22855780814606419, 37.50000000000000000 ) ) ;
#5550=PLANE ( 'NONE',  #11006 ) ;
#5553=( NAMED_UNIT ( * ) PLANE_ANGLE_UNIT ( ) SI_UNIT ( $, .RADIAN. ) );
#5564=VERTEX_POINT ( 'NONE', #15378 ) ;
#5579=DIRECTION ( 'NONE',  ( -1.000000000000000000, 0.000000000000000000, 0.000000000000000000 ) ) ;
#5622=ADVANCED_FACE ( 'NONE', ( #5900 ), #4332, .T. ) ;
#5689=AXIS2_PLACEMENT_3D ( 'NONE', #16260, #8887, #4944 ) ;
#5695=CIRCLE ( 'NONE', #4487, 7.168074330098680669 ) ;
#5722=EDGE_CURVE ( 'NONE', #6290, #715, #4153, .T. ) ;
#5763=EDGE_LOOP ( 'NONE', ( #18429, #14805, #17005, #3614 ) ) ;
#5779=VERTEX_POINT ( 'NONE', #14601 ) ;
#5781=CARTESIAN_POINT ( 'NONE',  ( 0.000000000000000000, 0.000000000000000000, 0.000000000000000000 ) ) ;
#5782=DIRECTION ( 'NONE',  ( 1.000000000000000000, 0.000000000000000000, 0.000000000000000000 ) ) ;
#5793=ORIENTED_EDGE ( 'NONE', *, *, #15805, .F. ) ;
#5805=CARTESIAN_POINT ( 'NONE',  ( -78.03414724812056136, 82.27553650601716129, 69.74547876954885339 ) ) ;
#5854=EDGE_CURVE ( 'NONE', #8416, #12329, #16666, .T. ) ;
#5884=ORIENTED_EDGE ( 'NONE', *, *, #17386, .F. ) ;
#5900=FACE_OUTER_BOUND ( 'NONE', #16304, .T. ) ;
#5914=ORIENTED_EDGE ( 'NONE', *, *, #3780, .T. ) ;
#5927=CARTESIAN_POINT ( 'NONE',  ( -57.08002265617300708, 84.22855780814606419, 68.73600986863397111 ) ) ;
#5938=CARTESIAN_POINT ( 'NONE',  ( -77.38579898953899772, 74.98691627113741731, 102.5000000000000000 ) ) ;
#5945=EDGE_CURVE ( 'NONE', #15227, #4300, #14306, .T. ) ;
#5947=CARTESIAN_POINT ( 'NONE',  ( -36.77424632280495587, 74.98691627113812785, 97.49999999999998579 ) ) ;
#5960=CARTESIAN_POINT ( 'NONE',  ( -37.41825604777831416, 91.72841893195356988, 62.00367782810642581 ) ) ;
#5972=DIRECTION ( 'NONE',  ( -0.000000000000000000, -0.000000000000000000, 1.000000000000000000 ) ) ;
#5984=DIRECTION ( 'NONE',  ( -1.000000000000000000, 0.000000000000000000, 0.000000000000000000 ) ) ;
#6023=CARTESIAN_POINT ( 'NONE',  ( -49.58002265617300708, 84.22855780814606419, -35.00000000000000000 ) ) ;
#6034=CARTESIAN_POINT ( 'NONE',  ( -106.3193689061042164, 112.6569076202650450, 97.49999999999998579 ) ) ;
#6037=DIRECTION ( 'NONE',  ( 0.000000000000000000, 0.000000000000000000, 1.000000000000000000 ) ) ;
#6038=CARTESIAN_POINT ( 'NONE',  ( -40.83486628351231218, 66.64375664990294013, 92.50000000000000000 ) ) ;
#6047=CARTESIAN_POINT ( 'NONE',  ( -36.20358435058752633, 86.88560906486404178, 55.48211817979245808 ) ) ;
#6059=ORIENTED_EDGE ( 'NONE', *, *, #2414, .T. ) ;
#6066=CARTESIAN_POINT ( 'NONE',  ( -78.12361985383351737, 83.98232705807352261, 55.00000000000002842 ) ) ;
#6079=CARTESIAN_POINT ( 'NONE',  ( -57.08002265617300708, 84.22855780814606419, 37.50000000000000000 ) ) ;
#6082=AXIS2_PLACEMENT_3D ( 'NONE', #1441, #32, #14446 ) ;
#6094=CYLINDRICAL_SURFACE ( 'NONE', #3959, 11.04359719766049430 ) ;
#6142=ORIENTED_EDGE ( 'NONE', *, *, #3410, .F. ) ;
#6147=CYLINDRICAL_SURFACE ( 'NONE', #15693, 7.500000000000000000 ) ;
#6156=EDGE_CURVE ( 'NONE', #17891, #8485, #16436, .T. ) ;
#6172=CARTESIAN_POINT ( 'NONE',  ( -38.09490121289055509, 73.26749283227019305, 97.49999999999998579 ) ) ;
#6178=CARTESIAN_POINT ( 'NONE',  ( -77.53403837096536222, 89.18782894963362651, 56.85235929646029263 ) ) ;
#6220=EDGE_CURVE ( 'NONE', #8703, #7660, #1978, .T. ) ;
#6237=DIRECTION ( 'NONE',  ( -0.000000000000000000, -0.000000000000000000, 1.000000000000000000 ) ) ;
#6241=CARTESIAN_POINT ( 'NONE',  ( -47.88253357122329845, 84.22855780814606419, 77.50000000000000000 ) ) ;
#6257=PRODUCT_DEFINITION_CONTEXT ( 'detailed design', #11001, 'design' ) ;
#6271=CARTESIAN_POINT ( 'NONE',  ( -78.08890555966455338, 85.46113186790836380, 55.09782012572272691 ) ) ;
#6281=ORIENTED_EDGE ( 'NONE', *, *, #2248, .F. ) ;
#6286=TOROIDAL_SURFACE ( 'NONE', #36, 47.49926016645015636, 5.000000000000000000 ) ;
#6290=VERTEX_POINT ( 'NONE', #1207 ) ;
#6333=AXIS2_PLACEMENT_3D ( 'NONE', #16741, #1238, #10032 ) ;
#6348=VECTOR ( 'NONE', #6912, 1000.000000000000000 ) ;
#6350=ORIENTED_EDGE ( 'NONE', *, *, #5351, .T. ) ;
#6379=EDGE_LOOP ( 'NONE', ( #15275, #3623, #4089, #5442 ) ) ;
#6380=PRODUCT ( 'High-Ratio Toggle Operating Handle', 'High-Ratio Toggle Operating Handle', '', ( #8278 ) ) ;
#6388=VERTEX_POINT ( 'NONE', #14222 ) ;
#6435=CARTESIAN_POINT ( 'NONE',  ( -37.14175463882769890, 77.49513323845337709, 65.84001190467381548 ) ) ;
#6438=CIRCLE ( 'NONE', #12128, 5.000000000000004441 ) ;
#6467=CARTESIAN_POINT ( 'NONE',  ( -76.76096363794077604, 91.67867170800820986, 61.50632582155040495 ) ) ;
#6513=ADVANCED_FACE ( 'NONE', ( #3030 ), #6286, .T. ) ;
#6520=CARTESIAN_POINT ( 'NONE',  ( -37.27023256319369438, 77.12848153769259341, 60.07106347578592676 ) ) ;
#6524=AXIS2_PLACEMENT_3D ( 'NONE', #11602, #9830, #718 ) ;
#6538=DIRECTION ( 'NONE',  ( -1.000000000000000000, 0.000000000000000000, 0.000000000000000000 ) ) ;
#6549=VECTOR ( 'NONE', #15762, 1000.000000000000000 ) ;
#6569=AXIS2_PLACEMENT_3D ( 'NONE', #4490, #17221, #1970 ) ;
#6585=CIRCLE ( 'NONE', #8990, 7.168074330098680669 ) ;
#6599=EDGE_CURVE ( 'NONE', #10149, #9739, #627, .T. ) ;
#6601=CARTESIAN_POINT ( 'NONE',  ( -76.76083043436963749, 76.77809071147591169, 61.50853494822962375 ) ) ;
#6619=CARTESIAN_POINT ( 'NONE',  ( -37.14248503629701048, 77.49305091727374872, 59.16519171840705127 ) ) ;
#6643=CIRCLE ( 'NONE', #10524, 2.168074330099287295 ) ;
#6661=LINE ( 'NONE', #9657, #9612 ) ;
#6688=ORIENTED_EDGE ( 'NONE', *, *, #1689, .T. ) ;
#6705=CARTESIAN_POINT ( 'NONE',  ( -78.08891603537360027, 82.99614312904147084, 55.09779029373265047 ) ) ;
#6714=CARTESIAN_POINT ( 'NONE',  ( -78.12361985383350316, 84.22855780814606419, 77.50000000000000000 ) ) ;
#6724=CARTESIAN_POINT ( 'NONE',  ( -36.04074584300169448, 83.73612801793909455, 69.98790387965719617 ) ) ;
#6757=DIRECTION ( 'NONE',  ( -1.000000000000000000, 0.000000000000000000, 0.000000000000000000 ) ) ;
#6762=CARTESIAN_POINT ( 'NONE',  ( -77.13858828394022282, 90.59309441108072747, 66.47525235387308840 ) ) ;
#6778=EDGE_CURVE ( 'NONE', #6388, #10149, #11976, .T. ) ;
#6789=ORIENTED_EDGE ( 'NONE', *, *, #8349, .F. ) ;
#6812=CARTESIAN_POINT ( 'NONE',  ( -36.03642545851251100, 84.22855780814606419, 70.00000000000001421 ) ) ;
#6834=AXIS2_PLACEMENT_3D ( 'NONE', #6079, #17862, #3194 ) ;
#6845=CIRCLE ( 'NONE', #12848, 11.04359719766049430 ) ;
#6848=CARTESIAN_POINT ( 'NONE',  ( -77.86214395528257626, 87.56725157785864155, 69.23390454379837422 ) ) ;
#6866=EDGE_CURVE ( 'NONE', #7744, #5248, #13205, .T. ) ;
#6880=DIRECTION ( 'NONE',  ( -0.9913829028483789330, -0.1309959539066817280, 0.000000000000000000 ) ) ;
#6905=DIRECTION ( 'NONE',  ( 0.7930648017909424086, 0.6091372753003162499, 5.105014369306161237E-16 ) ) ;
#6912=DIRECTION ( 'NONE',  ( -0.000000000000000000, -0.000000000000000000, -1.000000000000000000 ) ) ;
#6952=LINE ( 'NONE', #5065, #8378 ) ;
#6969=CIRCLE ( 'NONE', #13830, 2.168074330098676672 ) ;
#6974=DIRECTION ( 'NONE',  ( 1.000000000000000000, 0.000000000000000000, -0.000000000000000000 ) ) ;
#6975=FACE_OUTER_BOUND ( 'NONE', #16067, .T. ) ;
#6979=CARTESIAN_POINT ( 'NONE',  ( -49.58002265617300708, 84.22855780814606419, -35.00000000000000000 ) ) ;
#7022=FACE_OUTER_BOUND ( 'NONE', #12284, .T. ) ;
#7031=DIRECTION ( 'NONE',  ( -1.000000000000000000, 0.000000000000000000, 0.000000000000000000 ) ) ;
#7038=AXIS2_PLACEMENT_3D ( 'NONE', #16014, #11621, #13123 ) ;
#7064=( LENGTH_UNIT ( ) NAMED_UNIT ( * ) SI_UNIT ( .MILLI., .METRE. ) );
#7086=ORIENTED_EDGE ( 'NONE', *, *, #15403, .F. ) ;
#7098=CARTESIAN_POINT ( 'NONE',  ( -68.12361985383350316, 84.22855780814606419, 35.00000000000000000 ) ) ;
#7101=ORIENTED_EDGE ( 'NONE', *, *, #13741, .F. ) ;
#7159=CIRCLE ( 'NONE', #13124, 1.000000000000000888 ) ;
#7199=CARTESIAN_POINT ( 'NONE',  ( -76.06514409945376087, 73.26749283226919829, 97.49999999999998579 ) ) ;
#7217=DIRECTION ( 'NONE',  ( -0.000000000000000000, -0.000000000000000000, -1.000000000000000000 ) ) ;
#7220=DIRECTION ( 'NONE',  ( -1.000000000000000000, 0.000000000000000000, 0.000000000000000000 ) ) ;
#7251=EDGE_CURVE ( 'NONE', #2786, #2549, #2693, .T. ) ;
#7266=ORIENTED_EDGE ( 'NONE', *, *, #4038, .F. ) ;
#7273=ORIENTED_EDGE ( 'NONE', *, *, #6778, .T. ) ;
#7295=CARTESIAN_POINT ( 'NONE',  ( -37.27435264852402241, 91.34252568597628397, 64.92569797180529179 ) ) ;
#7300=DIRECTION ( 'NONE',  ( -0.000000000000000000, -0.000000000000000000, -1.000000000000000000 ) ) ;
#7303=ORIENTED_EDGE ( 'NONE', *, *, #5351, .F. ) ;
#7323=AXIS2_PLACEMENT_3D ( 'NONE', #16708, #1395, #2890 ) ;
#7364=EDGE_LOOP ( 'NONE', ( #5260, #6059, #13655, #5043 ) ) ;
#7382=CARTESIAN_POINT ( 'NONE',  ( -37.34514748644593851, 91.53406102980444814, 60.78507314490369140 ) ) ;
#7413=DIRECTION ( 'NONE',  ( -0.9240607556975078962, -0.3822456275482439825, -1.060944741915880422E-15 ) ) ;
#7416=DIRECTION ( 'NONE',  ( 0.000000000000000000, 0.000000000000000000, -1.000000000000000000 ) ) ;
#7418=ADVANCED_FACE ( 'NONE', ( #10349 ), #1735, .T. ) ;
#7419=DIRECTION ( 'NONE',  ( 1.000000000000000000, 0.000000000000000000, 0.000000000000000000 ) ) ;
#7428=LINE ( 'NONE', #11484, #11175 ) ;
#7432=CARTESIAN_POINT ( 'NONE',  ( -67.12361985383350316, 84.22855780814606419, -61.50000000000001421 ) ) ;
#7464=CARTESIAN_POINT ( 'NONE',  ( -36.53593263535576341, 88.80498052294456102, 56.53818285498137186 ) ) ;
#7486=AXIS2_PLACEMENT_3D ( 'NONE', #12156, #13650, #12058 ) ;
#7499=DIRECTION ( 'NONE',  ( -1.000000000000000000, 0.000000000000000000, 0.000000000000000000 ) ) ;
#7526=DIRECTION ( 'NONE',  ( -0.000000000000000000, -1.000000000000000000, -0.000000000000000000 ) ) ;
#7559=CARTESIAN_POINT ( 'NONE',  ( -36.07113975268146788, 85.46113186790836380, 69.90217987427729440 ) ) ;
#7570=CARTESIAN_POINT ( 'NONE',  ( -36.17543036020666136, 81.80210967128934385, 55.39904201915711468 ) ) ;
#7584=AXIS2_PLACEMENT_3D ( 'NONE', #3885, #2594, #9791 ) ;
#7593=ORIENTED_EDGE ( 'NONE', *, *, #13622, .T. ) ;
#7610=ORIENTED_EDGE ( 'NONE', *, *, #5133, .T. ) ;
#7614=DIRECTION ( 'NONE',  ( -0.000000000000000000, -0.000000000000000000, -1.000000000000000000 ) ) ;
#7660=VERTEX_POINT ( 'NONE', #4794 ) ;
#7702=ORIENTED_EDGE ( 'NONE', *, *, #2064, .T. ) ;
#7744=VERTEX_POINT ( 'NONE', #12688 ) ;
#7753=FACE_OUTER_BOUND ( 'NONE', #15590, .T. ) ;
#7759=AXIS2_PLACEMENT_3D ( 'NONE', #16951, #11344, #7220 ) ;
#7762=VERTEX_POINT ( 'NONE', #13985 ) ;
#7774=AXIS2_PLACEMENT_3D ( 'NONE', #12445, #12234, #17843 ) ;
#7787=DIRECTION ( 'NONE',  ( 0.000000000000000000, -1.000000000000000000, 0.000000000000000000 ) ) ;
#7792=ORIENTED_EDGE ( 'NONE', *, *, #9454, .F. ) ;
#7824=CARTESIAN_POINT ( 'NONE',  ( -54.93063083320800644, 106.4346967249107792, 102.5000000000000000 ) ) ;
#7850=CIRCLE ( 'NONE', #9048, 11.04359719766050141 ) ;
#7853=DIRECTION ( 'NONE',  ( 0.000000000000000000, 0.000000000000000000, 1.000000000000000000 ) ) ;
#7883=DIRECTION ( 'NONE',  ( -1.000000000000000000, 0.000000000000000000, 0.000000000000000000 ) ) ;
#7941=CARTESIAN_POINT ( 'NONE',  ( -37.32701571189549838, 76.97167339262615826, 64.45706195283406714 ) ) ;
#7949=CARTESIAN_POINT ( 'NONE',  ( -57.08002265617300708, 84.22855780814606419, -35.00000000000000000 ) ) ;
#7973=ORIENTED_EDGE ( 'NONE', *, *, #2778, .T. ) ;
#7986=CARTESIAN_POINT ( 'NONE',  ( -57.08002265617300708, 84.22855780814606419, -35.00000000000000000 ) ) ;
#8002=CARTESIAN_POINT ( 'NONE',  ( -77.98774719866210603, 81.79799583099486426, 55.38794294486089598 ) ) ;
#8020=CARTESIAN_POINT ( 'NONE',  ( -37.27426920733778104, 77.11479169650115750, 64.92672983002162823 ) ) ;
#8024=CARTESIAN_POINT ( 'NONE',  ( -33.72855994630469212, 78.95224028009285178, 102.5000000000000000 ) ) ;
#8034=ADVANCED_FACE ( 'NONE', ( #9100 ), #4545, .T. ) ;
#8056=CARTESIAN_POINT ( 'NONE',  ( -77.98770377200993664, 86.65978693925960386, 55.38805143041505374 ) ) ;
#8082=AXIS2_PLACEMENT_3D ( 'NONE', #12808, #14022, #9904 ) ;
#8086=DIRECTION ( 'NONE',  ( -0.000000000000000000, -0.000000000000000000, -1.000000000000000000 ) ) ;
#8089=EDGE_CURVE ( 'NONE', #13449, #8653, #6969, .T. ) ;
#8093=LINE ( 'NONE', #16510, #15326 ) ;
#8096=CARTESIAN_POINT ( 'NONE',  ( -77.26565842541029383, 78.27883601870418318, 57.92718427577206342 ) ) ;
#8114=DIRECTION ( 'NONE',  ( 0.000000000000000000, 0.000000000000000000, -1.000000000000000000 ) ) ;
#8116=CARTESIAN_POINT ( 'NONE',  ( -36.05803663064089903, 83.24379415027478046, 69.93918222302725951 ) ) ;
#8117=ORIENTED_EDGE ( 'NONE', *, *, #5854, .T. ) ;
#8124=VECTOR ( 'NONE', #17348, 1000.000000000000000 ) ;
#8160=EDGE_LOOP ( 'NONE', ( #6281, #6350, #2514, #16313, #8520 ) ) ;
#8163=CARTESIAN_POINT ( 'NONE',  ( -76.81489782590004722, 91.53406102980444814, 64.21492685509633702 ) ) ;
#8172=CIRCLE ( 'NONE', #7584, 4.999999999999997335 ) ;
#8189=EDGE_CURVE ( 'NONE', #3765, #11369, #7850, .T. ) ;
#8243=FACE_OUTER_BOUND ( 'NONE', #18005, .T. ) ;
#8244=AXIS2_PLACEMENT_3D ( 'NONE', #10828, #4939, #13729 ) ;
#8278=PRODUCT_CONTEXT ( 'NONE', #9803, 'mechanical' ) ;
#8298=CARTESIAN_POINT ( 'NONE',  ( -78.23321842955243710, 73.26749283226919829, 102.5000000000000000 ) ) ;
#8341=CARTESIAN_POINT ( 'NONE',  ( -57.08002265617300708, 84.22855780814606419, -35.00000000000000000 ) ) ;
#8349=EDGE_CURVE ( 'NONE', #4147, #16002, #1872, .T. ) ;
#8359=ORIENTED_EDGE ( 'NONE', *, *, #10867, .T. ) ;
#8364=CARTESIAN_POINT ( 'NONE',  ( -40.83486628351231218, 66.64375664990294013, 102.5000000000000000 ) ) ;
#8370=DIRECTION ( 'NONE',  ( -0.000000000000000000, -0.000000000000000000, -1.000000000000000000 ) ) ;
#8378=VECTOR ( 'NONE', #10783, 1000.000000000000000 ) ;
#8409=CARTESIAN_POINT ( 'NONE',  ( -64.58002265617299997, 84.22855780814606419, 35.00000000000000000 ) ) ;
#8412=ORIENTED_EDGE ( 'NONE', *, *, #5722, .F. ) ;
#8416=VERTEX_POINT ( 'NONE', #3165 ) ;
#8443=CARTESIAN_POINT ( 'NONE',  ( -91.19225650277898865, 92.96220022626712876, 92.50000000000000000 ) ) ;
#8454=VERTEX_POINT ( 'NONE', #6038 ) ;
#8466=CARTESIAN_POINT ( 'NONE',  ( -33.72855994630469212, 78.95224028009285178, 92.50000000000000000 ) ) ;
#8485=VERTEX_POINT ( 'NONE', #7824 ) ;
#8491=ORIENTED_EDGE ( 'NONE', *, *, #5273, .T. ) ;
#8499=DIRECTION ( 'NONE',  ( 1.000000000000000000, 0.000000000000000000, 0.000000000000000000 ) ) ;
#8520=ORIENTED_EDGE ( 'NONE', *, *, #15457, .T. ) ;
#8545=CARTESIAN_POINT ( 'NONE',  ( -78.12361985383348895, 83.72858089318386021, 70.00000000000002842 ) ) ;
#8587=DIRECTION ( 'NONE',  ( -1.000000000000000000, 0.000000000000000000, 0.000000000000000000 ) ) ;
#8603=ADVANCED_FACE ( 'NONE', ( #9600 ), #11468, .T. ) ;
#8645=DIRECTION ( 'NONE',  ( -0.000000000000000000, -0.000000000000000000, -1.000000000000000000 ) ) ;
#8653=VERTEX_POINT ( 'NONE', #8298 ) ;
#8668=CARTESIAN_POINT ( 'NONE',  ( -64.58002265617299997, 84.22855780814606419, -35.00000000000000000 ) ) ;
#8677=ORIENTED_EDGE ( 'NONE', *, *, #15664, .F. ) ;
#8678=AXIS2_PLACEMENT_3D ( 'NONE', #1495, #17212, #2991 ) ;
#8703=VERTEX_POINT ( 'NONE', #11919 ) ;
#8746=FACE_BOUND ( 'NONE', #641, .T. ) ;
#8758=DIRECTION ( 'NONE',  ( -0.000000000000000000, -0.000000000000000000, -1.000000000000000000 ) ) ;
#8786=ORIENTED_EDGE ( 'NONE', *, *, #4562, .F. ) ;
#8793=CARTESIAN_POINT ( 'NONE',  ( -37.39908167440526654, 91.67867170800822407, 63.49367417844965900 ) ) ;
#8825=TOROIDAL_SURFACE ( 'NONE', #155, 2.168074330098863189, 5.000000000000000000 ) ;
#8835=AXIS2_PLACEMENT_3D ( 'NONE', #2484, #8086, #9493 ) ;
#8848=DIRECTION ( 'NONE',  ( -0.000000000000000000, -0.000000000000000000, -1.000000000000000000 ) ) ;
#8855=CARTESIAN_POINT ( 'NONE',  ( -123.4618227840623632, 84.22855780814606419, 62.50000000000001421 ) ) ;
#8857=CARTESIAN_POINT ( 'NONE',  ( -49.97371631896665178, 107.0896764944441202, 92.50000000000000000 ) ) ;
#8868=VERTEX_POINT ( 'NONE', #3497 ) ;
#8883=CARTESIAN_POINT ( 'NONE',  ( -37.02145702840577712, 90.59309441108072747, 58.52474764612693292 ) ) ;
#8887=DIRECTION ( 'NONE',  ( -0.000000000000000000, -0.000000000000000000, -1.000000000000000000 ) ) ;
#8894=CARTESIAN_POINT ( 'NONE',  ( -77.35462390582623016, 78.58944219063714343, 57.54922146810498873 ) ) ;
#8907=EDGE_CURVE ( 'NONE', #8868, #14712, #9592, .T. ) ;
#8920=CARTESIAN_POINT ( 'NONE',  ( -78.12361985383350316, 84.22855780814606419, 77.50000000000000000 ) ) ;
#8958=VECTOR ( 'NONE', #12473, 1000.000000000000000 ) ;
#8961=DIRECTION ( 'NONE',  ( 1.000000000000000000, 0.000000000000000000, 0.000000000000000000 ) ) ;
#8967=CARTESIAN_POINT ( 'NONE',  ( -66.27751174112272281, 84.22855780814606419, 92.50000000000000000 ) ) ;
#8969=CARTESIAN_POINT ( 'NONE',  ( -36.05421503597830224, 85.21903647478332289, 55.04951438993911239 ) ) ;
#8984=CARTESIAN_POINT ( 'NONE',  ( -76.76056308706507991, 76.77737988954069692, 63.48723832607239359 ) ) ;
#8990=AXIS2_PLACEMENT_3D ( 'NONE', #15599, #2597, #896 ) ;
#9005=CYLINDRICAL_SURFACE ( 'NONE', #7038, 9.197489084949710403 ) ;
#9013=CARTESIAN_POINT ( 'NONE',  ( -75.23640716657462235, 71.26406042838958399, 102.5000000000000000 ) ) ;
#9048=AXIS2_PLACEMENT_3D ( 'NONE', #8341, #14053, #5782 ) ;
#9064=CARTESIAN_POINT ( 'NONE',  ( -36.03642545851253232, 84.72841810161554577, 55.00000000000002842 ) ) ;
#9069=EDGE_CURVE ( 'NONE', #10128, #5779, #17963, .T. ) ;
#9071=CIRCLE ( 'NONE', #2195, 21.04359719766049608 ) ;
#9083=AXIS2_PLACEMENT_3D ( 'NONE', #12582, #2467, #11075 ) ;
#9100=FACE_OUTER_BOUND ( 'NONE', #10237, .T. ) ;
#9101=STYLED_ITEM('',(#18573),#314);
#9113=CYLINDRICAL_SURFACE ( 'NONE', #9245, 11.04359719766049430 ) ;
#9152=DIRECTION ( 'NONE',  ( -1.000000000000000000, 2.693970411862685384E-15, 0.000000000000000000 ) ) ;
#9156=ADVANCED_FACE ( 'NONE', ( #16952, #3943 ), #18368, .T. ) ;
#9177=DIRECTION ( 'NONE',  ( -1.000000000000000000, 6.400974180244839938E-15, 0.000000000000000000 ) ) ;
#9237=EDGE_CURVE ( 'NONE', #715, #7744, #6661, .T. ) ;
#9243=VERTEX_POINT ( 'NONE', #1241 ) ;
#9245=AXIS2_PLACEMENT_3D ( 'NONE', #14804, #9292, #1994 ) ;
#9251=DIRECTION ( 'NONE',  ( 1.000000000000000000, 0.000000000000000000, 0.000000000000000000 ) ) ;
#9275=AXIS2_PLACEMENT_3D ( 'NONE', #2408, #8114, #17930 ) ;
#9285=CARTESIAN_POINT ( 'NONE',  ( -57.08002265617300708, 84.22855780814606419, 35.00000000000000000 ) ) ;
#9287=CARTESIAN_POINT ( 'NONE',  ( -77.09746718839080870, 90.72084218871722783, 58.73700743486453746 ) ) ;
#9292=DIRECTION ( 'NONE',  ( 0.000000000000000000, 0.000000000000000000, -1.000000000000000000 ) ) ;
#9315=CIRCLE ( 'NONE', #15610, 2.168074330098864078 ) ;
#9324=CARTESIAN_POINT ( 'NONE',  ( -76.91951136665340982, 77.21161119120515082, 65.15931570389709293 ) ) ;
#9361=EDGE_LOOP ( 'NONE', ( #17811, #10538, #2670, #15288 ) ) ;
#9363=DIRECTION ( 'NONE',  ( 0.000000000000000000, 0.000000000000000000, 1.000000000000000000 ) ) ;
#9405=ORIENTED_EDGE ( 'NONE', *, *, #9069, .T. ) ;
#9438=CARTESIAN_POINT ( 'NONE',  ( -36.62711323603792124, 79.27386099610184544, 56.86433512711490579 ) ) ;
#9442=DIRECTION ( 'NONE',  ( 0.000000000000000000, 0.000000000000000000, 1.000000000000000000 ) ) ;
#9454=EDGE_CURVE ( 'NONE', #15032, #15460, #16161, .T. ) ;
#9466=DIRECTION ( 'NONE',  ( -0.000000000000000000, -0.000000000000000000, -1.000000000000000000 ) ) ;
#9472=ORIENTED_EDGE ( 'NONE', *, *, #2010, .F. ) ;
#9474=ORIENTED_EDGE ( 'NONE', *, *, #2248, .T. ) ;
#9490=DIRECTION ( 'NONE',  ( 0.000000000000000000, 0.000000000000000000, 1.000000000000000000 ) ) ;
#9493=DIRECTION ( 'NONE',  ( -1.000000000000000000, 0.000000000000000000, 0.000000000000000000 ) ) ;
#9506=CARTESIAN_POINT ( 'NONE',  ( -76.81489084760232799, 76.92303621577350725, 64.21479655795450014 ) ) ;
#9516=EDGE_CURVE ( 'NONE', #8485, #4505, #9315, .T. ) ;
#9522=CARTESIAN_POINT ( 'NONE',  ( -36.89537005233415812, 78.27079066365615745, 57.91772688325330876 ) ) ;
#9528=CYLINDRICAL_SURFACE ( 'NONE', #9717, 42.49926016644912607 ) ;
#9548=CIRCLE ( 'NONE', #16105, 11.04359719766050141 ) ;
#9592=CIRCLE ( 'NONE', #11697, 21.04359719766049608 ) ;
#9594=DIRECTION ( 'NONE',  ( 0.1309959539064320944, 0.9913829028484121286, 1.514972713530672604E-13 ) ) ;
#9600=FACE_OUTER_BOUND ( 'NONE', #10463, .T. ) ;
#9612=VECTOR ( 'NONE', #12383, 1000.000000000000000 ) ;
#9616=CARTESIAN_POINT ( 'NONE',  ( -36.53717731224358545, 79.64648582715004466, 68.45756564509078146 ) ) ;
#9620=AXIS2_PLACEMENT_3D ( 'NONE', #13155, #14639, #8587 ) ;
#9647=ORIENTED_EDGE ( 'NONE', *, *, #9069, .F. ) ;
#9657=CARTESIAN_POINT ( 'NONE',  ( -46.03642545851250389, 84.22855780814606419, 68.73600986863397111 ) ) ;
#9661=CARTESIAN_POINT ( 'NONE',  ( -77.78773836288226562, 87.99602245404173573, 69.00331597549191542 ) ) ;
#9692=DIRECTION ( 'NONE',  ( -0.1309959539066819501, 0.9913829028483791550, 0.000000000000000000 ) ) ;
#9717=AXIS2_PLACEMENT_3D ( 'NONE', #15231, #12745, #10268 ) ;
#9723=CARTESIAN_POINT ( 'NONE',  ( -37.39921487797633404, 76.77809071147591169, 63.49146505177037625 ) ) ;
#9739=VERTEX_POINT ( 'NONE', #267 ) ;
#9769=ORIENTED_EDGE ( 'NONE', *, *, #8349, .T. ) ;
#9791=DIRECTION ( 'NONE',  ( -1.000000000000000000, 0.000000000000000000, 0.000000000000000000 ) ) ;
#9803=APPLICATION_CONTEXT ( 'automotive_design' ) ;
#9830=DIRECTION ( 'NONE',  ( 0.000000000000000000, 0.000000000000000000, 1.000000000000000000 ) ) ;
#9860=CARTESIAN_POINT ( 'NONE',  ( -57.08002265617300708, 84.22855780814606419, -62.50000000000000000 ) ) ;
#9894=DIRECTION ( 'NONE',  ( 0.000000000000000000, 0.000000000000000000, 1.000000000000000000 ) ) ;
#9904=DIRECTION ( 'NONE',  ( -1.000000000000000000, 0.000000000000000000, 0.000000000000000000 ) ) ;
#9975=AXIS2_PLACEMENT_3D ( 'NONE', #15970, #17539, #3239 ) ;
#9995=DIRECTION ( 'NONE',  ( -0.000000000000000000, -0.000000000000000000, 1.000000000000000000 ) ) ;
#10002=DIRECTION ( 'NONE',  ( -0.000000000000000000, -0.000000000000000000, -1.000000000000000000 ) ) ;
#10010=EDGE_LOOP ( 'NONE', ( #13259, #2499, #4036, #10375 ) ) ;
#10032=DIRECTION ( 'NONE',  ( 1.000000000000000000, 0.000000000000000000, 0.000000000000000000 ) ) ;
#10057=DIRECTION ( 'NONE',  ( -0.000000000000000000, -0.000000000000000000, -1.000000000000000000 ) ) ;
#10060=CARTESIAN_POINT ( 'NONE',  ( -36.03642545851251100, 84.22855780814606419, 77.50000000000000000 ) ) ;
#10105=CARTESIAN_POINT ( 'NONE',  ( -36.62600694138065904, 89.18782894963364072, 68.14764070353975001 ) ) ;
#10128=VERTEX_POINT ( 'NONE', #4426 ) ;
#10130=AXIS2_PLACEMENT_3D ( 'NONE', #15156, #2340, #1341 ) ;
#10138=DIRECTION ( 'NONE',  ( -0.000000000000000000, -0.000000000000000000, -1.000000000000000000 ) ) ;
#10149=VERTEX_POINT ( 'NONE', #9013 ) ;
#10169=CIRCLE ( 'NONE', #6569, 7.168074330099288183 ) ;
#10177=EDGE_CURVE ( 'NONE', #14012, #14712, #1801, .T. ) ;
#10188=CARTESIAN_POINT ( 'NONE',  ( -57.08002265617300708, 84.22855780814606419, 77.50000000000000000 ) ) ;
#10191=CARTESIAN_POINT ( 'NONE',  ( -38.09490121289055509, 73.26749283227019305, 102.5000000000000000 ) ) ;
#10194=ADVANCED_FACE ( 'NONE', ( #17596 ), #6094, .T. ) ;
#10237=EDGE_LOOP ( 'NONE', ( #11433, #12213, #7303, #17229 ) ) ;
#10246=FACE_OUTER_BOUND ( 'NONE', #15086, .T. ) ;
#10253=CIRCLE ( 'NONE', #2181, 42.49926016645017057 ) ;
#10264=AXIS2_PLACEMENT_3D ( 'NONE', #16896, #9594, #14198 ) ;
#10268=DIRECTION ( 'NONE',  ( -1.000000000000000000, 0.000000000000000000, 0.000000000000000000 ) ) ;
#10278=CARTESIAN_POINT ( 'NONE',  ( -37.17496177488503406, 91.05728076224789902, 59.38899799626690168 ) ) ;
#10283=ORIENTED_EDGE ( 'NONE', *, *, #8189, .F. ) ;
#10297=CARTESIAN_POINT ( 'NONE',  ( -76.88577610500824733, 77.11479169650115750, 60.07327016997842151 ) ) ;
#10302=EDGE_LOOP ( 'NONE', ( #13881, #12546, #4928, #17510 ) ) ;
#10316=ORIENTED_EDGE ( 'NONE', *, *, #9516, .F. ) ;
#10326=AXIS2_PLACEMENT_3D ( 'NONE', #7199, #12822, #7031 ) ;
#10330=CARTESIAN_POINT ( 'NONE',  ( -36.03642545851251100, 84.22855780814606419, 77.50000000000000000 ) ) ;
#10349=FACE_OUTER_BOUND ( 'NONE', #5421, .T. ) ;
#10368=DIRECTION ( 'NONE',  ( 0.000000000000000000, 0.000000000000000000, 1.000000000000000000 ) ) ;
#10371=FACE_OUTER_BOUND ( 'NONE', #2747, .T. ) ;
#10374=CARTESIAN_POINT ( 'NONE',  ( -36.03642545851251811, 83.72858089318386021, 55.00000000000002132 ) ) ;
#10375=ORIENTED_EDGE ( 'NONE', *, *, #15664, .T. ) ;
#10394=ORIENTED_EDGE ( 'NONE', *, *, #13828, .T. ) ;
#10415=DIRECTION ( 'NONE',  ( 1.000000000000000000, -0.000000000000000000, -0.000000000000000000 ) ) ;
#10416=ORIENTED_EDGE ( 'NONE', *, *, #3410, .T. ) ;
#10440=ORIENTED_EDGE ( 'NONE', *, *, #2010, .T. ) ;
#10446=( LENGTH_UNIT ( ) NAMED_UNIT ( * ) SI_UNIT ( .MILLI., .METRE. ) );
#10453=CARTESIAN_POINT ( 'NONE',  ( -36.80510220921193820, 89.87539756129703505, 57.54020390674075713 ) ) ;
#10463=EDGE_LOOP ( 'NONE', ( #7086, #5793, #5914, #1788 ) ) ;
#10489=ORIENTED_EDGE ( 'NONE', *, *, #2657, .F. ) ;
#10494=CARTESIAN_POINT ( 'NONE',  ( -77.78632074013589204, 88.00379445693184266, 56.00117480735330133 ) ) ;
#10514=DIRECTION ( 'NONE',  ( 1.000000000000000000, 0.000000000000000000, 0.000000000000000000 ) ) ;
#10524=AXIS2_PLACEMENT_3D ( 'NONE', #3973, #13999, #1180 ) ;
#10538=ORIENTED_EDGE ( 'NONE', *, *, #4038, .T. ) ;
#10543=( NAMED_UNIT ( * ) PLANE_ANGLE_UNIT ( ) SI_UNIT ( $, .RADIAN. ) );
#10553=ORIENTED_EDGE ( 'NONE', *, *, #17960, .F. ) ;
#10595=( GEOMETRIC_REPRESENTATION_CONTEXT ( 3 ) GLOBAL_UNCERTAINTY_ASSIGNED_CONTEXT ( ( #851 ) ) GLOBAL_UNIT_ASSIGNED_CONTEXT ( ( #7064, #5553, #11074 ) ) REPRESENTATION_CONTEXT ( 'NONE', 'WORKASPACE' ) );
#10613=CIRCLE ( 'NONE', #4931, 42.49926016644946003 ) ;
#10649=ADVANCED_FACE ( 'NONE', ( #11973 ), #17409, .T. ) ;
#10658=EDGE_LOOP ( 'NONE', ( #9769, #3571 ) ) ;
#10672=DIRECTION ( 'NONE',  ( -0.000000000000000000, -0.000000000000000000, -1.000000000000000000 ) ) ;
#10690=CARTESIAN_POINT ( 'NONE',  ( -66.27751174112272281, 84.22855780814606419, 92.50000000000000000 ) ) ;
#10692=CARTESIAN_POINT ( 'NONE',  ( -38.09490121289055509, 73.26749283227019305, 97.49999999999998579 ) ) ;
#10698=AXIS2_PLACEMENT_3D ( 'NONE', #1252, #12680, #15170 ) ;
#10705=EDGE_LOOP ( 'NONE', ( #9472, #3752, #16875, #10953 ) ) ;
#10719=CARTESIAN_POINT ( 'NONE',  ( -77.78732798123100167, 80.45864980048332882, 69.00206661717221834 ) ) ;
#10756=EDGE_CURVE ( 'NONE', #16002, #12329, #8093, .T. ) ;
#10758=CARTESIAN_POINT ( 'NONE',  ( -57.08002265617301418, 106.1506877598988154, 102.5000000000000000 ) ) ;
#10783=DIRECTION ( 'NONE',  ( 1.000000000000000000, -0.000000000000000000, -0.000000000000000000 ) ) ;
#10811=ORIENTED_EDGE ( 'NONE', *, *, #14930, .F. ) ;
#10812=ORIENTED_EDGE ( 'NONE', *, *, #7251, .T. ) ;
#10817=CARTESIAN_POINT ( 'NONE',  ( -77.62069601435324273, 79.65130292775347698, 68.44629942221835961 ) ) ;
#10828=CARTESIAN_POINT ( 'NONE',  ( -57.08002265617300708, 84.22855780814606419, 77.50000000000000000 ) ) ;
#10834=CARTESIAN_POINT ( 'NONE',  ( -36.37271733111500538, 80.45864980048332882, 55.99793338282779587 ) ) ;
#10840=VERTEX_POINT ( 'NONE', #3712 ) ;
#10867=EDGE_CURVE ( 'NONE', #2786, #10840, #9071, .T. ) ;
#10877=CARTESIAN_POINT ( 'NONE',  ( -78.12361985383350316, 84.22855780814606419, 55.00000000000001421 ) ) ;
#10920=VERTEX_POINT ( 'NONE', #18493 ) ;
#10926=CARTESIAN_POINT ( 'NONE',  ( -76.83752720176745754, 76.98425793134822470, 64.45727744071827203 ) ) ;
#10935=ORIENTED_EDGE ( 'NONE', *, *, #16227, .F. ) ;
#10940=CARTESIAN_POINT ( 'NONE',  ( -36.30023241575587178, 80.89962780276930232, 69.22524214366039530 ) ) ;
#10953=ORIENTED_EDGE ( 'NONE', *, *, #14331, .F. ) ;
#10958=CARTESIAN_POINT ( 'NONE',  ( -57.08002265617300708, 84.22855780814606419, 77.50000000000000000 ) ) ;
#10968=CARTESIAN_POINT ( 'NONE',  ( -49.97371631896665178, 107.0896764944441202, 97.49999999999998579 ) ) ;
#10973=CARTESIAN_POINT ( 'NONE',  ( -78.10583027636772613, 85.21903647478332289, 69.95048561006090893 ) ) ;
#10998=ORIENTED_EDGE ( 'NONE', *, *, #3456, .F. ) ;
#11001=APPLICATION_CONTEXT ( 'automotive_design' ) ;
#11006=AXIS2_PLACEMENT_3D ( 'NONE', #15556, #12487, #4148 ) ;
#11027=CARTESIAN_POINT ( 'NONE',  ( -37.24053394569259723, 77.21161119120516503, 59.84068429610289286 ) ) ;
#11032=ORIENTED_EDGE ( 'NONE', *, *, #7251, .F. ) ;
#11064=CARTESIAN_POINT ( 'NONE',  ( -77.09753311995068259, 90.72064142110008333, 66.26335585294400232 ) ) ;
#11074=( NAMED_UNIT ( * ) SI_UNIT ( $, .STERADIAN. ) SOLID_ANGLE_UNIT ( ) );
#11075=DIRECTION ( 'NONE',  ( 1.000000000000000000, 0.000000000000000000, 0.000000000000000000 ) ) ;
#11087=ADVANCED_FACE ( 'NONE', ( #11642 ), #14365, .F. ) ;
#11123=AXIS2_PLACEMENT_3D ( 'NONE', #17690, #3480, #13590 ) ;
#11140=DIRECTION ( 'NONE',  ( -0.000000000000000000, -0.000000000000000000, 1.000000000000000000 ) ) ;
#11173=PRODUCT_DEFINITION_FORMATION_WITH_SPECIFIED_SOURCE ( 'ANY', '', #6380, .NOT_KNOWN. ) ;
#11175=VECTOR ( 'NONE', #8758, 1000.000000000000000 ) ;
#11226=CARTESIAN_POINT ( 'NONE',  ( -77.38579898953862823, 74.98691627113693414, 97.49999999999998579 ) ) ;
#11268=ORIENTED_EDGE ( 'NONE', *, *, #1689, .F. ) ;
#11321=AXIS2_PLACEMENT_3D ( 'NONE', #10692, #7614, #11911 ) ;
#11344=DIRECTION ( 'NONE',  ( -1.224646799147353207E-16, 1.000000000000000000, 0.000000000000000000 ) ) ;
#11358=ORIENTED_EDGE ( 'NONE', *, *, #13741, .T. ) ;
#11367=ORIENTED_EDGE ( 'NONE', *, *, #17960, .T. ) ;
#11369=VERTEX_POINT ( 'NONE', #4299 ) ;
#11390=VERTEX_POINT ( 'NONE', #350 ) ;
#11391=VECTOR ( 'NONE', #12991, 1000.000000000000000 ) ;
#11433=ORIENTED_EDGE ( 'NONE', *, *, #17733, .F. ) ;
#11465=DIRECTION ( 'NONE',  ( -1.000000000000000000, 0.000000000000000000, 0.000000000000000000 ) ) ;
#11468=TOROIDAL_SURFACE ( 'NONE', #4867, 10.04359719766049963, 1.000000000000000000 ) ;
#11484=CARTESIAN_POINT ( 'NONE',  ( -49.97371631896665178, 107.0896764944441202, 102.5000000000000000 ) ) ;
#11500=CYLINDRICAL_SURFACE ( 'NONE', #8082, 42.49926016644946003 ) ;
#11530=CIRCLE ( 'NONE', #3431, 5.000000000000004441 ) ;
#11540=ORIENTED_EDGE ( 'NONE', *, *, #10867, .F. ) ;
#11569=ORIENTED_EDGE ( 'NONE', *, *, #12149, .T. ) ;
#11574=ORIENTED_EDGE ( 'NONE', *, *, #16689, .F. ) ;
#11602=CARTESIAN_POINT ( 'NONE',  ( -7.840676406241780860, 112.6569076202650308, 97.49999999999998579 ) ) ;
#11605=AXIS2_PLACEMENT_3D ( 'NONE', #4699, #10415, #14709 ) ;
#11621=DIRECTION ( 'NONE',  ( -0.000000000000000000, -0.000000000000000000, -1.000000000000000000 ) ) ;
#11628=CARTESIAN_POINT ( 'NONE',  ( -57.08002265617302839, 27.37185818390810965, 102.5000000000000000 ) ) ;
#11629=CARTESIAN_POINT ( 'NONE',  ( -57.08002265617300708, 84.22855780814606419, -35.00000000000000000 ) ) ;
#11642=FACE_OUTER_BOUND ( 'NONE', #4510, .T. ) ;
#11683=CARTESIAN_POINT ( 'NONE',  ( -37.27023353548769791, 91.32863676353444760, 60.07107215585045878 ) ) ;
#11686=VECTOR ( 'NONE', #10057, 1000.000000000000000 ) ;
#11687=EDGE_CURVE ( 'NONE', #315, #13818, #14756, .T. ) ;
#11697=AXIS2_PLACEMENT_3D ( 'NONE', #12302, #598, #10514 ) ;
#11771=DIRECTION ( 'NONE',  ( -0.000000000000000000, -0.000000000000000000, -1.000000000000000000 ) ) ;
#11774=CARTESIAN_POINT ( 'NONE',  ( -36.17496312660223623, 86.65089956811803518, 55.39766986458640474 ) ) ;
#11795=CARTESIAN_POINT ( 'NONE',  ( -76.83302960045048735, 76.97167339262611563, 60.54293804716597549 ) ) ;
#11801=ORIENTED_EDGE ( 'NONE', *, *, #16710, .T. ) ;
#11835=DIRECTION ( 'NONE',  ( 1.000000000000000000, -0.000000000000000000, -0.000000000000000000 ) ) ;
#11837=DIRECTION ( 'NONE',  ( 0.000000000000000000, 0.000000000000000000, -1.000000000000000000 ) ) ;
#11853=SHAPE_REPRESENTATION_RELATIONSHIP ( 'NONE' , 'NONE' ,  #14258, #13725 ) ;
#11861=CARTESIAN_POINT ( 'NONE',  ( -36.80651802494987379, 89.88064937530403142, 67.45419788538286809 ) ) ;
#11911=DIRECTION ( 'NONE',  ( -1.000000000000000000, 0.000000000000000000, 0.000000000000000000 ) ) ;
#11919=CARTESIAN_POINT ( 'NONE',  ( -36.03642545851251100, 84.22855780814606419, 55.00000000000001421 ) ) ;
#11925=AXIS2_PLACEMENT_3D ( 'NONE', #17599, #4976, #7883 ) ;
#11944=ORIENTED_EDGE ( 'NONE', *, *, #5034, .F. ) ;
#11973=FACE_OUTER_BOUND ( 'NONE', #12883, .T. ) ;
#11976=CIRCLE ( 'NONE', #3915, 5.000000000000006217 ) ;
#11981=CIRCLE ( 'NONE', #3921, 47.49926016645014926 ) ;
#11987=DIRECTION ( 'NONE',  ( -1.000000000000000000, 6.400974180245392929E-15, 0.000000000000000000 ) ) ;
#12028=CIRCLE ( 'NONE', #6333, 21.04359719766049608 ) ;
#12058=DIRECTION ( 'NONE',  ( 1.000000000000000000, 0.000000000000000000, -0.000000000000000000 ) ) ;
#12075=B_SPLINE_CURVE_WITH_KNOTS ( 'NONE', 3,
 ( #10877, #5062, #861, #17795, #6271, #16380, #8056, #14801, #10494, #3569, #6178, #17594, #4776, #16193, #9287, #3383, #13595, #779, #1991, #6467, #12187, #17878, #2453, #8163, #12387, #16655, #12568, #16751, #5341, #11064, #6762, #13877, #1070, #3948, #13970, #9661, #6848, #964, #12480, #18172, #15370, #10973, #18082, #2563 ),
 .UNSPECIFIED., .F., .F.,
 ( 4, 2, 2, 2, 2, 2, 2, 2, 2, 2, 2, 2, 2, 2, 2, 2, 2, 2, 2, 2, 2, 4 ),
 ( 0.02364448373982101781, 0.02438320150779627049, 0.02512191927577152317, 0.02659935481172202854, 0.02807679034767253390, 0.02955422588362303926, 0.03103166141957354116, 0.03177037918754879731, 0.03250909695552404999, 0.03398653249147452760, 0.03546396802742500520, 0.03694140356337549669, 0.03768012133135077019, 0.03841883909932603675, 0.03915755686730131024, 0.03989627463527657680, 0.04137371017122713768, 0.04285114570717769855, 0.04432858124312825249, 0.04506729901110352599, 0.04580601677907880642, 0.04728345231502940199 ),
 .UNSPECIFIED. ) ;
#12081=MECHANICAL_DESIGN_GEOMETRIC_PRESENTATION_REPRESENTATION('',(#9101),#10595);
#12128=AXIS2_PLACEMENT_3D ( 'NONE', #2169, #7787, #15164 ) ;
#12149=EDGE_CURVE ( 'NONE', #17012, #15227, #18085, .T. ) ;
#12156=CARTESIAN_POINT ( 'NONE',  ( -57.08002265617300708, 84.22855780814606419, 37.50000000000000000 ) ) ;
#12167=DIRECTION ( 'NONE',  ( 1.000000000000000000, 0.000000000000000000, 0.000000000000000000 ) ) ;
#12168=VERTEX_POINT ( 'NONE', #8466 ) ;
#12187=CARTESIAN_POINT ( 'NONE',  ( -76.74168354031206718, 91.72869609463793950, 62.00788389762995223 ) ) ;
#12197=CIRCLE ( 'NONE', #4423, 5.000000000000007994 ) ;
#12213=ORIENTED_EDGE ( 'NONE', *, *, #2746, .T. ) ;
#12219=CARTESIAN_POINT ( 'NONE',  ( -77.62286800010241450, 79.64648582715007308, 56.54243435490922565 ) ) ;
#12234=DIRECTION ( 'NONE',  ( -0.000000000000000000, -0.000000000000000000, -1.000000000000000000 ) ) ;
#12236=CARTESIAN_POINT ( 'NONE',  ( -36.62539116635755931, 79.27196096192943742, 68.14973479026978964 ) ) ;
#12270=ADVANCED_FACE ( 'NONE', ( #7753 ), #8825, .T. ) ;
#12284=EDGE_LOOP ( 'NONE', ( #4167, #13967, #9474, #10394 ) ) ;
#12302=CARTESIAN_POINT ( 'NONE',  ( -57.08002265617300708, 84.22855780814606419, 37.50000000000000000 ) ) ;
#12326=CARTESIAN_POINT ( 'NONE',  ( -77.95601046370802578, 81.56801578385646678, 69.51654028185745915 ) ) ;
#12329=VERTEX_POINT ( 'NONE', #6241 ) ;
#12343=CARTESIAN_POINT ( 'NONE',  ( -36.80542140651982663, 78.58944219063717185, 67.45077853189506811 ) ) ;
#12355=DIRECTION ( 'NONE',  ( -0.000000000000000000, -0.000000000000000000, -1.000000000000000000 ) ) ;
#12383=DIRECTION ( 'NONE',  ( 0.000000000000000000, 0.000000000000000000, -1.000000000000000000 ) ) ;
#12387=CARTESIAN_POINT ( 'NONE',  ( -76.83752798444122334, 91.47285552305426393, 64.45728441025069344 ) ) ;
#12414=EDGE_LOOP ( 'NONE', ( #148, #15574, #4011, #13315 ) ) ;
#12429=CARTESIAN_POINT ( 'NONE',  ( -78.03761615004539465, 82.26638713947221504, 55.24423648577771218 ) ) ;
#12445=CARTESIAN_POINT ( 'NONE',  ( -76.06514409945376087, 73.26749283226919829, 97.49999999999998579 ) ) ;
#12468=UNCERTAINTY_MEASURE_WITH_UNIT (LENGTH_MEASURE( 1.000000000000000082E-05 ), #10446, 'distance_accuracy_value', 'NONE');
#12473=DIRECTION ( 'NONE',  ( 0.000000000000000000, 0.000000000000000000, -1.000000000000000000 ) ) ;
#12477=EDGE_CURVE ( 'NONE', #14712, #8868, #449, .T. ) ;
#12480=CARTESIAN_POINT ( 'NONE',  ( -77.98508218574379214, 86.65089956811806360, 69.60233013541360947 ) ) ;
#12487=DIRECTION ( 'NONE',  ( -0.000000000000000000, 0.000000000000000000, -1.000000000000000000 ) ) ;
#12496=EDGE_LOOP ( 'NONE', ( #554, #10283 ) ) ;
#12505=EDGE_LOOP ( 'NONE', ( #3883, #5024 ) ) ;
#12517=ORIENTED_EDGE ( 'NONE', *, *, #335, .T. ) ;
#12522=EDGE_LOOP ( 'NONE', ( #3924, #18469, #8786, #5884 ) ) ;
#12533=CARTESIAN_POINT ( 'NONE',  ( -36.12242916230060530, 82.26638713947218662, 69.75576351422232335 ) ) ;
#12546=ORIENTED_EDGE ( 'NONE', *, *, #8189, .T. ) ;
#12568=CARTESIAN_POINT ( 'NONE',  ( -76.91954306033080968, 91.24541864506342392, 65.15959670748108579 ) ) ;
#12579=ADVANCED_FACE ( 'NONE', ( #13095 ), #4356, .T. ) ;
#12582=CARTESIAN_POINT ( 'NONE',  ( -57.08002265617300708, 84.22855780814606419, -35.00000000000000000 ) ) ;
#12604=AXIS2_PLACEMENT_3D ( 'NONE', #11628, #14179, #18479 ) ;
#12609=CIRCLE ( 'NONE', #634, 7.500000000000000000 ) ;
#12610=EDGE_CURVE ( 'NONE', #4147, #8416, #14924, .T. ) ;
#12626=DIRECTION ( 'NONE',  ( -0.000000000000000000, -0.000000000000000000, -1.000000000000000000 ) ) ;
#12633=DIRECTION ( 'NONE',  ( -0.6091372753003161389, 0.7930648017909424086, 0.000000000000000000 ) ) ;
#12680=DIRECTION ( 'NONE',  ( -0.000000000000000000, -0.000000000000000000, -1.000000000000000000 ) ) ;
#12688=CARTESIAN_POINT ( 'NONE',  ( -46.03642545851250389, 84.22855780814606419, 35.00000000000000000 ) ) ;
#12698=CIRCLE ( 'NONE', #125, 7.168074330099291736 ) ;
#12700=DIRECTION ( 'NONE',  ( -0.000000000000000000, -0.000000000000000000, -1.000000000000000000 ) ) ;
#12712=EDGE_CURVE ( 'NONE', #3765, #15435, #356, .T. ) ;
#12714=EDGE_CURVE ( 'NONE', #15151, #6388, #10613, .T. ) ;
#12720=ORIENTED_EDGE ( 'NONE', *, *, #14331, .T. ) ;
#12742=VECTOR ( 'NONE', #1853, 1000.000000000000000 ) ;
#12745=DIRECTION ( 'NONE',  ( -0.000000000000000000, -0.000000000000000000, -1.000000000000000000 ) ) ;
#12761=CARTESIAN_POINT ( 'NONE',  ( -46.03642545851250389, 84.22855780814606419, 37.50000000000000000 ) ) ;
#12785=FACE_OUTER_BOUND ( 'NONE', #12496, .T. ) ;
#12808=CARTESIAN_POINT ( 'NONE',  ( -57.08002265617302839, 27.37185818390810965, 102.5000000000000000 ) ) ;
#12822=DIRECTION ( 'NONE',  ( -0.000000000000000000, -0.000000000000000000, -1.000000000000000000 ) ) ;
#12848=AXIS2_PLACEMENT_3D ( 'NONE', #15818, #5972, #3095 ) ;
#12878=VECTOR ( 'NONE', #15809, 1000.000000000000000 ) ;
#12883=EDGE_LOOP ( 'NONE', ( #4494, #14386, #7101, #18239 ) ) ;
#12891=CARTESIAN_POINT ( 'NONE',  ( -57.08002265617300708, 84.22855780814606419, -61.50000000000001421 ) ) ;
#12918=AXIS2_PLACEMENT_3D ( 'NONE', #17856, #7853, #12167 ) ;
#12928=DIRECTION ( 'NONE',  ( 0.000000000000000000, 0.000000000000000000, 1.000000000000000000 ) ) ;
#12941=CARTESIAN_POINT ( 'NONE',  ( -46.03642545851250389, 84.22855780814606419, -61.50000000000001421 ) ) ;
#12991=DIRECTION ( 'NONE',  ( -0.000000000000000000, -0.000000000000000000, -1.000000000000000000 ) ) ;
#12995=CLOSED_SHELL ( 'NONE', ( #14404, #4130, #2893, #15117, #8034, #17785, #361, #11087, #3759, #15903, #2938, #4998, #14402, #4150, #5398, #7418, #14532, #5622, #14544, #14309, #1186, #13991, #5508, #9156, #13377, #5481, #12579, #10649, #6513, #12270, #16694, #3893, #918, #2400, #8603, #10194 ) ) ;
#13011=CARTESIAN_POINT ( 'NONE',  ( -57.08002265617300708, 84.22855780814606419, 77.50000000000000000 ) ) ;
#13034=ORIENTED_EDGE ( 'NONE', *, *, #6220, .F. ) ;
#13079=LINE ( 'NONE', #8668, #18257 ) ;
#13087=ORIENTED_EDGE ( 'NONE', *, *, #6599, .T. ) ;
#13095=FACE_OUTER_BOUND ( 'NONE', #10705, .T. ) ;
#13097=CARTESIAN_POINT ( 'NONE',  ( -37.32251732790476950, 91.47285552305426393, 60.54271558974930656 ) ) ;
#13099=ORIENTED_EDGE ( 'NONE', *, *, #16449, .F. ) ;
#13120=DIRECTION ( 'NONE',  ( -0.000000000000000000, -0.000000000000000000, -1.000000000000000000 ) ) ;
#13123=DIRECTION ( 'NONE',  ( -1.000000000000000000, 0.000000000000000000, 0.000000000000000000 ) ) ;
#13124=AXIS2_PLACEMENT_3D ( 'NONE', #7432, #7526, #11837 ) ;
#13148=AXIS2_PLACEMENT_3D ( 'NONE', #14952, #17574, #17671 ) ;
#13151=ORIENTED_EDGE ( 'NONE', *, *, #5133, .F. ) ;
#13155=CARTESIAN_POINT ( 'NONE',  ( -57.08002265617300708, 84.22855780814606419, 92.50000000000000000 ) ) ;
#13184=CARTESIAN_POINT ( 'NONE',  ( -36.29766045040744160, 87.56553636334628266, 69.23463151675950655 ) ) ;
#13198=CARTESIAN_POINT ( 'NONE',  ( -78.11929946934434099, 83.73612801793909455, 55.01209612034283936 ) ) ;
#13205=CIRCLE ( 'NONE', #4808, 11.04359719766050141 ) ;
#13214=EDGE_CURVE ( 'NONE', #12329, #8416, #13577, .T. ) ;
#13220=EDGE_LOOP ( 'NONE', ( #3746, #10440, #10811, #7273 ) ) ;
#13239=AXIS2_PLACEMENT_3D ( 'NONE', #4824, #4725, #17639 ) ;
#13259=ORIENTED_EDGE ( 'NONE', *, *, #2911, .F. ) ;
#13260=DIRECTION ( 'NONE',  ( -0.7930648017910726377, 0.6091372753001467188, 0.000000000000000000 ) ) ;
#13273=CARTESIAN_POINT ( 'NONE',  ( -36.53760766897426038, 88.81248391902217065, 68.45606934554520251 ) ) ;
#13276=CARTESIAN_POINT ( 'NONE',  ( -76.06514409945376087, 73.26749283226919829, 92.50000000000000000 ) ) ;
#13280=CARTESIAN_POINT ( 'NONE',  ( -36.20403484863803101, 81.56801578385648099, 55.48345971814259769 ) ) ;
#13284=AXIS2_PLACEMENT_3D ( 'NONE', #9860, #2749, #7499 ) ;
#13314=DIRECTION ( 'NONE',  ( -1.000000000000000000, 0.000000000000000000, 0.000000000000000000 ) ) ;
#13315=ORIENTED_EDGE ( 'NONE', *, *, #3214, .F. ) ;
#13358=CARTESIAN_POINT ( 'NONE',  ( -36.03642545851251100, 84.47473112397162254, 70.00000000000002842 ) ) ;
#13377=ADVANCED_FACE ( 'NONE', ( #18228 ), #13893, .T. ) ;
#13420=DIRECTION ( 'NONE',  ( 1.000000000000000000, 0.000000000000000000, 0.000000000000000000 ) ) ;
#13425=ORIENTED_EDGE ( 'NONE', *, *, #10177, .T. ) ;
#13449=VERTEX_POINT ( 'NONE', #5938 ) ;
#13528=CARTESIAN_POINT ( 'NONE',  ( -38.09490121289055509, 73.26749283227019305, 102.5000000000000000 ) ) ;
#13537=AXIS2_PLACEMENT_3D ( 'NONE', #17670, #10672, #6538 ) ;
#13554=CARTESIAN_POINT ( 'NONE',  ( -36.03642545851251100, 83.98232705807349419, 70.00000000000002842 ) ) ;
#13577=CIRCLE ( 'NONE', #8244, 9.197489084949710403 ) ;
#13586=CARTESIAN_POINT ( 'NONE',  ( -76.06514409945376087, 73.26749283226919829, 102.5000000000000000 ) ) ;
#13590=DIRECTION ( 'NONE',  ( -1.000000000000000000, 0.000000000000000000, 0.000000000000000000 ) ) ;
#13595=CARTESIAN_POINT ( 'NONE',  ( -76.98456221794718601, 91.05880801963004956, 59.39221631177008476 ) ) ;
#13614=ORIENTED_EDGE ( 'NONE', *, *, #12149, .F. ) ;
#13622=EDGE_CURVE ( 'NONE', #9739, #5564, #18063, .T. ) ;
#13650=DIRECTION ( 'NONE',  ( 0.000000000000000000, 0.000000000000000000, 1.000000000000000000 ) ) ;
#13651=CARTESIAN_POINT ( 'NONE',  ( -36.07112927697242100, 82.99614312904145663, 69.90220970626739927 ) ) ;
#13653=EDGE_LOOP ( 'NONE', ( #15716, #17579, #11801, #16339, #981, #13087, #7593, #4455 ) ) ;
#13655=ORIENTED_EDGE ( 'NONE', *, *, #16227, .T. ) ;
#13659=CARTESIAN_POINT ( 'NONE',  ( -57.08002265617302839, 27.37185818390810965, 92.50000000000000000 ) ) ;
#13704=EDGE_LOOP ( 'NONE', ( #3040, #17691, #10416, #970 ) ) ;
#13725=ADVANCED_BREP_SHAPE_REPRESENTATION ( '', ( #314, #16217 ), #2194 ) ;
#13729=DIRECTION ( 'NONE',  ( 1.000000000000000000, 0.000000000000000000, 0.000000000000000000 ) ) ;
#13733=CARTESIAN_POINT ( 'NONE',  ( -36.26589399568750594, 81.12099773066753983, 69.33028675349314085 ) ) ;
#13741=EDGE_CURVE ( 'NONE', #8485, #15227, #11530, .T. ) ;
#13815=CARTESIAN_POINT ( 'NONE',  ( -77.78561374552398888, 80.46558623543624833, 56.00764281523724009 ) ) ;
#13818=VERTEX_POINT ( 'NONE', #6979 ) ;
#13828=EDGE_CURVE ( 'NONE', #12168, #15032, #3155, .T. ) ;
#13830=AXIS2_PLACEMENT_3D ( 'NONE', #13586, #17870, #11987 ) ;
#13836=CIRCLE ( 'NONE', #3373, 4.999999999999993783 ) ;
#13856=DIRECTION ( 'NONE',  ( -1.000000000000000000, 0.000000000000000000, 0.000000000000000000 ) ) ;
#13871=FACE_OUTER_BOUND ( 'NONE', #13220, .T. ) ;
#13877=CARTESIAN_POINT ( 'NONE',  ( -77.26539832087783566, 90.18382313193714594, 67.08526386498388661 ) ) ;
#13881=ORIENTED_EDGE ( 'NONE', *, *, #12712, .F. ) ;
#13893=TOROIDAL_SURFACE ( 'NONE', #7323, 47.49926016644946003, 5.000000000000000000 ) ;
#13932=DIRECTION ( 'NONE',  ( -0.000000000000000000, -0.000000000000000000, -1.000000000000000000 ) ) ;
#13949=ORIENTED_EDGE ( 'NONE', *, *, #4353, .F. ) ;
#13967=ORIENTED_EDGE ( 'NONE', *, *, #5945, .T. ) ;
#13970=CARTESIAN_POINT ( 'NONE',  ( -77.62411267699025075, 88.80498052294456102, 68.46181714501862814 ) ) ;
#13985=CARTESIAN_POINT ( 'NONE',  ( -80.43148536604020649, 78.95224028009165806, 92.50000000000000000 ) ) ;
#13986=ORIENTED_EDGE ( 'NONE', *, *, #6220, .T. ) ;
#13991=ADVANCED_FACE ( 'NONE', ( #8243 ), #16362, .T. ) ;
#13999=DIRECTION ( 'NONE',  ( 0.000000000000000000, 0.000000000000000000, 1.000000000000000000 ) ) ;
#14004=CIRCLE ( 'NONE', #11321, 7.168074330099291736 ) ;
#14012=VERTEX_POINT ( 'NONE', #17956 ) ;
#14022=DIRECTION ( 'NONE',  ( -0.000000000000000000, -0.000000000000000000, -1.000000000000000000 ) ) ;
#14053=DIRECTION ( 'NONE',  ( -0.000000000000000000, -0.000000000000000000, -1.000000000000000000 ) ) ;
#14079=ORIENTED_EDGE ( 'NONE', *, *, #4562, .T. ) ;
#14179=DIRECTION ( 'NONE',  ( -0.000000000000000000, -0.000000000000000000, -1.000000000000000000 ) ) ;
#14198=DIRECTION ( 'NONE',  ( -0.9913829028484120176, 0.1309959539064320944, 0.000000000000000000 ) ) ;
#14204=DIRECTION ( 'NONE',  ( 0.000000000000000000, 0.000000000000000000, -1.000000000000000000 ) ) ;
#14205=EDGE_CURVE ( 'NONE', #14448, #18509, #17334, .T. ) ;
#14218=EDGE_CURVE ( 'NONE', #6290, #5248, #1228, .T. ) ;
#14220=DIRECTION ( 'NONE',  ( -1.000000000000000000, 0.000000000000000000, 0.000000000000000000 ) ) ;
#14222=CARTESIAN_POINT ( 'NONE',  ( -73.32517902883354566, 66.64375664990241432, 97.49999999999998579 ) ) ;
#14233=CARTESIAN_POINT ( 'NONE',  ( -57.08002265617300708, 84.22855780814606419, -61.50000000000001421 ) ) ;
#14249=CARTESIAN_POINT ( 'NONE',  ( -78.05508519719376181, 82.51445519007735641, 69.80563559789565886 ) ) ;
#14258=SHAPE_REPRESENTATION ( 'High-Ratio Toggle Operating Handle', ( #16217 ), #2194 ) ;
#14260=ORIENTED_EDGE ( 'NONE', *, *, #8907, .F. ) ;
#14306=CIRCLE ( 'NONE', #6524, 42.49926016644912607 ) ;
#14309=ADVANCED_FACE ( 'NONE', ( #14762 ), #1589, .T. ) ;
#14331=EDGE_CURVE ( 'NONE', #11390, #10920, #3281, .T. ) ;
#14352=CARTESIAN_POINT ( 'NONE',  ( -57.08002265617300708, 84.22855780814606419, 68.73600986863397111 ) ) ;
#14353=ORIENTED_EDGE ( 'NONE', *, *, #6866, .T. ) ;
#14365=CYLINDRICAL_SURFACE ( 'NONE', #4584, 7.500000000000000000 ) ;
#14386=ORIENTED_EDGE ( 'NONE', *, *, #5945, .F. ) ;
#14388=DIRECTION ( 'NONE',  ( -0.6091372753001471629, -0.7930648017910721936, 0.000000000000000000 ) ) ;
#14402=ADVANCED_FACE ( 'NONE', ( #16529, #14931 ), #18035, .F. ) ;
#14404=ADVANCED_FACE ( 'NONE', ( #15223 ), #18137, .T. ) ;
#14441=ORIENTED_EDGE ( 'NONE', *, *, #2414, .F. ) ;
#14444=CIRCLE ( 'NONE', #3682, 2.168074330098676672 ) ;
#14446=DIRECTION ( 'NONE',  ( -1.000000000000000000, 0.000000000000000000, 0.000000000000000000 ) ) ;
#14448=VERTEX_POINT ( 'NONE', #8409 ) ;
#14466=CYLINDRICAL_SURFACE ( 'NONE', #17296, 11.04359719766049430 ) ;
#14532=ADVANCED_FACE ( 'NONE', ( #18332 ), #4292, .F. ) ;
#14534=DIRECTION ( 'NONE',  ( 0.000000000000000000, 0.000000000000000000, 1.000000000000000000 ) ) ;
#14544=ADVANCED_FACE ( 'NONE', ( #5403 ), #11500, .F. ) ;
#14572=FACE_OUTER_BOUND ( 'NONE', #16266, .T. ) ;
#14576=CARTESIAN_POINT ( 'NONE',  ( -36.89464699146818560, 90.18382313193718858, 57.91473613501618445 ) ) ;
#14585=TOROIDAL_SURFACE ( 'NONE', #10698, 2.168074330099288183, 5.000000000000000000 ) ;
#14601=CARTESIAN_POINT ( 'NONE',  ( -47.03642545851250389, 84.22855780814606419, -62.50000000000000000 ) ) ;
#14622=TOROIDAL_SURFACE ( 'NONE', #3564, 2.168074330098679336, 5.000000000000000000 ) ;
#14629=CARTESIAN_POINT ( 'NONE',  ( -46.03642545851250389, 84.22855780814606419, -35.00000000000000000 ) ) ;
#14639=DIRECTION ( 'NONE',  ( -0.000000000000000000, -0.000000000000000000, -1.000000000000000000 ) ) ;
#14648=CIRCLE ( 'NONE', #8678, 9.197489084949710403 ) ;
#14663=CARTESIAN_POINT ( 'NONE',  ( -36.12242140784905331, 86.19059744224306030, 69.75578550468861749 ) ) ;
#14669=CARTESIAN_POINT ( 'NONE',  ( -36.10496011515223103, 82.51445519007735641, 55.19436440210437667 ) ) ;
#14670=ORIENTED_EDGE ( 'NONE', *, *, #4239, .T. ) ;
#14677=CARTESIAN_POINT ( 'NONE',  ( -77.53465414598844063, 79.27196096192940900, 56.85026520973028141 ) ) ;
#14679=CARTESIAN_POINT ( 'NONE',  ( -64.18632899337946185, 107.0896764944433954, 92.50000000000000000 ) ) ;
#14702=CARTESIAN_POINT ( 'NONE',  ( -75.23640716657477867, 71.26406042838995347, 97.49999999999998579 ) ) ;
#14709=DIRECTION ( 'NONE',  ( 0.000000000000000000, 0.000000000000000000, -1.000000000000000000 ) ) ;
#14712=VERTEX_POINT ( 'NONE', #3059 ) ;
#14751=CARTESIAN_POINT ( 'NONE',  ( -36.03642545851251100, 84.22855780814606419, 55.00000000000001421 ) ) ;
#14756=CIRCLE ( 'NONE', #3724, 7.500000000000000000 ) ;
#14762=FACE_OUTER_BOUND ( 'NONE', #8160, .T. ) ;
#14795=VECTOR ( 'NONE', #16246, 1000.000000000000000 ) ;
#14801=CARTESIAN_POINT ( 'NONE',  ( -77.86238486193855124, 87.56553636334633950, 55.76536848324052897 ) ) ;
#14804=CARTESIAN_POINT ( 'NONE',  ( -57.08002265617300708, 84.22855780814606419, 68.73600986863397111 ) ) ;
#14805=ORIENTED_EDGE ( 'NONE', *, *, #11687, .T. ) ;
#14907=AXIS2_PLACEMENT_3D ( 'NONE', #1729, #15698, #18495 ) ;
#14921=ORIENTED_EDGE ( 'NONE', *, *, #12610, .F. ) ;
#14924=LINE ( 'NONE', #8967, #12742 ) ;
#14926=ORIENTED_EDGE ( 'NONE', *, *, #6778, .F. ) ;
#14930=EDGE_CURVE ( 'NONE', #6388, #11390, #6585, .T. ) ;
#14931=FACE_OUTER_BOUND ( 'NONE', #4720, .T. ) ;
#14952=CARTESIAN_POINT ( 'NONE',  ( -57.08002265617300708, 84.22855780814606419, 35.00000000000000000 ) ) ;
#14997=EDGE_CURVE ( 'NONE', #7762, #9243, #592, .T. ) ;
#15020=CARTESIAN_POINT ( 'NONE',  ( -76.74163717699387632, 76.72829797731421309, 62.01011918307220583 ) ) ;
#15032=VERTEX_POINT ( 'NONE', #8857 ) ;
#15036=CARTESIAN_POINT ( 'NONE',  ( -36.53934929799278564, 79.65130292775349119, 56.55370057778164750 ) ) ;
#15038=AXIS2_PLACEMENT_3D ( 'NONE', #874, #4703, #16111 ) ;
#15068=CARTESIAN_POINT ( 'NONE',  ( -36.77424632280495587, 74.98691627113812785, 102.5000000000000000 ) ) ;
#15086=EDGE_LOOP ( 'NONE', ( #1066, #18233, #13151, #3819 ) ) ;
#15117=ADVANCED_FACE ( 'NONE', ( #13871 ), #14622, .T. ) ;
#15119=CARTESIAN_POINT ( 'NONE',  ( -77.48836037079389882, 79.09395985567564935, 67.97217490261259343 ) ) ;
#15132=CARTESIAN_POINT ( 'NONE',  ( -37.39948222528091293, 76.77737988954068271, 61.51276167392764194 ) ) ;
#15151=VERTEX_POINT ( 'NONE', #2343 ) ;
#15156=CARTESIAN_POINT ( 'NONE',  ( -106.3193689061042164, 112.6569076202650450, 92.50000000000000000 ) ) ;
#15164=DIRECTION ( 'NONE',  ( 0.000000000000000000, 0.000000000000000000, -1.000000000000000000 ) ) ;
#15167=CARTESIAN_POINT ( 'NONE',  ( -68.12361985383350316, 84.22855780814606419, -61.50000000000001421 ) ) ;
#15170=DIRECTION ( 'NONE',  ( -1.000000000000000000, 0.000000000000000000, 0.000000000000000000 ) ) ;
#15172=EDGE_CURVE ( 'NONE', #11369, #4264, #3760, .T. ) ;
#15197=VERTEX_POINT ( 'NONE', #16470 ) ;
#15203=CARTESIAN_POINT ( 'NONE',  ( -76.88981274915232689, 77.12848153769257920, 64.92893652421413719 ) ) ;
#15223=FACE_OUTER_BOUND ( 'NONE', #13704, .T. ) ;
#15224=CARTESIAN_POINT ( 'NONE',  ( -36.93791207748871841, 78.13360439242255495, 66.87729283127455915 ) ) ;
#15226=AXIS2_PLACEMENT_3D ( 'NONE', #2586, #9490, #6974 ) ;
#15227=VERTEX_POINT ( 'NONE', #10968 ) ;
#15228=CIRCLE ( 'NONE', #7759, 1.000000000000000888 ) ;
#15231=CARTESIAN_POINT ( 'NONE',  ( -7.840676406241780860, 112.6569076202650308, 102.5000000000000000 ) ) ;
#15254=AXIS2_PLACEMENT_3D ( 'NONE', #5502, #10002, #14220 ) ;
#15275=ORIENTED_EDGE ( 'NONE', *, *, #4239, .F. ) ;
#15288=ORIENTED_EDGE ( 'NONE', *, *, #6866, .F. ) ;
#15289=FACE_BOUND ( 'NONE', #1071, .T. ) ;
#15320=CARTESIAN_POINT ( 'NONE',  ( -36.17229811368392944, 81.79799583099489269, 69.61205705513911823 ) ) ;
#15326=VECTOR ( 'NONE', #3800, 1000.000000000000000 ) ;
#15370=CARTESIAN_POINT ( 'NONE',  ( -78.05523331206480009, 85.94077383471115184, 69.80605996636154487 ) ) ;
#15378=CARTESIAN_POINT ( 'NONE',  ( -35.92682688279126779, 73.26749283227019305, 102.5000000000000000 ) ) ;
#15384=DIRECTION ( 'NONE',  ( -0.000000000000000000, -0.000000000000000000, -1.000000000000000000 ) ) ;
#15403=EDGE_CURVE ( 'NONE', #15435, #5779, #15228, .T. ) ;
#15435=VERTEX_POINT ( 'NONE', #12941 ) ;
#15457=EDGE_CURVE ( 'NONE', #8454, #12168, #10169, .T. ) ;
#15460=VERTEX_POINT ( 'NONE', #14679 ) ;
#15529=VECTOR ( 'NONE', #16100, 1000.000000000000000 ) ;
#15556=CARTESIAN_POINT ( 'NONE',  ( -91.19225650277898865, 92.96220022626712876, 102.5000000000000000 ) ) ;
#15574=ORIENTED_EDGE ( 'NONE', *, *, #13622, .F. ) ;
#15590=EDGE_LOOP ( 'NONE', ( #11358, #13614, #5003, #10316 ) ) ;
#15599=CARTESIAN_POINT ( 'NONE',  ( -76.06514409945376087, 73.26749283226919829, 97.49999999999998579 ) ) ;
#15610=AXIS2_PLACEMENT_3D ( 'NONE', #16274, #3463, #9177 ) ;
#15647=CARTESIAN_POINT ( 'NONE',  ( -78.12361985383350316, 84.22855780814607840, 70.00000000000001421 ) ) ;
#15664=EDGE_CURVE ( 'NONE', #2078, #8454, #17036, .T. ) ;
#15682=EDGE_CURVE ( 'NONE', #11369, #3765, #15847, .T. ) ;
#15693=AXIS2_PLACEMENT_3D ( 'NONE', #16438, #6237, #9251 ) ;
#15698=DIRECTION ( 'NONE',  ( 0.000000000000000000, 0.000000000000000000, 1.000000000000000000 ) ) ;
#15716=ORIENTED_EDGE ( 'NONE', *, *, #6156, .T. ) ;
#15722=VECTOR ( 'NONE', #11771, 1000.000000000000000 ) ;
#15759=DIRECTION ( 'NONE',  ( 1.000000000000000000, 0.000000000000000000, -0.000000000000000000 ) ) ;
#15762=DIRECTION ( 'NONE',  ( -0.000000000000000000, -0.000000000000000000, -1.000000000000000000 ) ) ;
#15784=AXIS2_PLACEMENT_3D ( 'NONE', #1354, #13120, #5984 ) ;
#15798=ORIENTED_EDGE ( 'NONE', *, *, #11687, .F. ) ;
#15804=CARTESIAN_POINT ( 'NONE',  ( -37.06257812395524098, 90.72084218871721362, 66.26299256513551938 ) ) ;
#15805=EDGE_CURVE ( 'NONE', #4264, #15435, #5383, .T. ) ;
#15809=DIRECTION ( 'NONE',  ( 0.000000000000000000, 0.000000000000000000, -1.000000000000000000 ) ) ;
#15818=CARTESIAN_POINT ( 'NONE',  ( -57.08002265617300708, 84.22855780814606419, -61.50000000000001421 ) ) ;
#15847=CIRCLE ( 'NONE', #604, 11.04359719766050141 ) ;
#15887=CARTESIAN_POINT ( 'NONE',  ( -36.17234154033610594, 86.65978693925961807, 69.61194856958498178 ) ) ;
#15903=ADVANCED_FACE ( 'NONE', ( #14572 ), #264, .T. ) ;
#15952=CIRCLE ( 'NONE', #10130, 42.49926016645017057 ) ;
#15970=CARTESIAN_POINT ( 'NONE',  ( -57.08002265617300708, 84.22855780814606419, -62.50000000000000000 ) ) ;
#15983=CARTESIAN_POINT ( 'NONE',  ( -37.13915117359674412, 90.95236025322212470, 59.16826207617363309 ) ) ;
#15990=AXIS2_PLACEMENT_3D ( 'NONE', #10758, #3750, #13856 ) ;
#16002=VERTEX_POINT ( 'NONE', #2026 ) ;
#16014=CARTESIAN_POINT ( 'NONE',  ( -57.08002265617300708, 84.22855780814606419, 92.50000000000000000 ) ) ;
#16023=CARTESIAN_POINT ( 'NONE',  ( -106.3193689061042164, 112.6569076202650450, 102.5000000000000000 ) ) ;
#16049=PLANE ( 'NONE',  #9975 ) ;
#16057=LINE ( 'NONE', #3336, #15722 ) ;
#16060=CARTESIAN_POINT ( 'NONE',  ( -36.10481200028119275, 85.94077383471113762, 55.19394003363846224 ) ) ;
#16063=DIRECTION ( 'NONE',  ( -1.000000000000000000, 0.000000000000000000, 0.000000000000000000 ) ) ;
#16067=EDGE_LOOP ( 'NONE', ( #1537, #6688, #3980, #16582 ) ) ;
#16072=CARTESIAN_POINT ( 'NONE',  ( -78.10200868170512933, 83.24379415027480889, 55.06081777697277602 ) ) ;
#16080=CARTESIAN_POINT ( 'NONE',  ( -59.22941447913701296, 106.4346967249104239, 102.5000000000000000 ) ) ;
#16098=DIRECTION ( 'NONE',  ( -0.000000000000000000, -0.000000000000000000, -1.000000000000000000 ) ) ;
#16100=DIRECTION ( 'NONE',  ( 1.000000000000000000, -0.000000000000000000, -0.000000000000000000 ) ) ;
#16105=AXIS2_PLACEMENT_3D ( 'NONE', #3136, #8848, #7419 ) ;
#16111=DIRECTION ( 'NONE',  ( 0.3822456275483139820, 0.9240607556974786974, 0.000000000000000000 ) ) ;
#16139=( NAMED_UNIT ( * ) SI_UNIT ( $, .STERADIAN. ) SOLID_ANGLE_UNIT ( ) );
#16148=CARTESIAN_POINT ( 'NONE',  ( -36.62604544348833713, 89.18779308299876618, 56.85266771181889567 ) ) ;
#16161=CIRCLE ( 'NONE', #12918, 7.168074330098860969 ) ;
#16166=DIRECTION ( 'NONE',  ( -1.000000000000000000, 0.000000000000000000, 0.000000000000000000 ) ) ;
#16193=CARTESIAN_POINT ( 'NONE',  ( -77.13785763070544022, 90.59536451873515261, 58.52851757989075310 ) ) ;
#16210=ORIENTED_EDGE ( 'NONE', *, *, #10756, .T. ) ;
#16217=AXIS2_PLACEMENT_3D ( 'NONE', #5781, #6037, #8961 ) ;
#16227=EDGE_CURVE ( 'NONE', #17012, #15460, #18418, .T. ) ;
#16234=CARTESIAN_POINT ( 'NONE',  ( -78.12361985383350316, 84.22855780814607840, 70.00000000000001421 ) ) ;
#16237=ORIENTED_EDGE ( 'NONE', *, *, #10177, .F. ) ;
#16245=EDGE_CURVE ( 'NONE', #315, #14448, #13079, .T. ) ;
#16246=DIRECTION ( 'NONE',  ( 0.000000000000000000, 0.000000000000000000, -1.000000000000000000 ) ) ;
#16260=CARTESIAN_POINT ( 'NONE',  ( -7.840676406241780860, 112.6569076202650308, 102.5000000000000000 ) ) ;
#16266=EDGE_LOOP ( 'NONE', ( #10553, #5171, #3013, #2092, #1095, #16237, #7702, #11032 ) ) ;
#16269=FACE_OUTER_BOUND ( 'NONE', #5763, .T. ) ;
#16274=CARTESIAN_POINT ( 'NONE',  ( -57.08002265617301418, 106.1506877598988154, 102.5000000000000000 ) ) ;
#16275=ORIENTED_EDGE ( 'NONE', *, *, #6599, .F. ) ;
#16304=EDGE_LOOP ( 'NONE', ( #11268, #12720, #17519, #17321 ) ) ;
#16313=ORIENTED_EDGE ( 'NONE', *, *, #2911, .T. ) ;
#16339=ORIENTED_EDGE ( 'NONE', *, *, #8089, .T. ) ;
#16362=CYLINDRICAL_SURFACE ( 'NONE', #15990, 7.168074330098860969 ) ;
#16368=ORIENTED_EDGE ( 'NONE', *, *, #15457, .F. ) ;
#16380=CARTESIAN_POINT ( 'NONE',  ( -78.03762390449695374, 86.19059744224304609, 55.24421449531139672 ) ) ;
#16415=CARTESIAN_POINT ( 'NONE',  ( -77.26467526001188446, 78.27079066365617166, 67.08227311674674809 ) ) ;
#16430=AXIS2_PLACEMENT_3D ( 'NONE', #13011, #17367, #1672 ) ;
#16436=CIRCLE ( 'NONE', #5689, 47.49926016644912607 ) ;
#16438=CARTESIAN_POINT ( 'NONE',  ( -57.08002265617300708, 84.22855780814606419, -35.00000000000000000 ) ) ;
#16440=AXIS2_PLACEMENT_3D ( 'NONE', #16622, #13932, #5309 ) ;
#16449=EDGE_CURVE ( 'NONE', #13818, #315, #12609, .T. ) ;
#16470=CARTESIAN_POINT ( 'NONE',  ( -30.92682688279126424, 73.26749283227019305, 97.49999999999998579 ) ) ;
#16479=ORIENTED_EDGE ( 'NONE', *, *, #9454, .T. ) ;
#16501=EDGE_LOOP ( 'NONE', ( #9405, #12517 ) ) ;
#16510=CARTESIAN_POINT ( 'NONE',  ( -47.88253357122329845, 84.22855780814606419, 92.50000000000000000 ) ) ;
#16515=CARTESIAN_POINT ( 'NONE',  ( -78.12361985383350316, 84.22855780814606419, 55.00000000000001421 ) ) ;
#16529=FACE_BOUND ( 'NONE', #3366, .T. ) ;
#16531=CARTESIAN_POINT ( 'NONE',  ( -37.41840813535210941, 76.72829797731419887, 62.98988081692781549 ) ) ;
#16535=DIRECTION ( 'NONE',  ( -1.000000000000000000, 0.000000000000000000, 0.000000000000000000 ) ) ;
#16582=ORIENTED_EDGE ( 'NONE', *, *, #1052, .F. ) ;
#16611=CARTESIAN_POINT ( 'NONE',  ( -77.40008690996572227, 78.75501449464320558, 57.36680777008252363 ) ) ;
#16622=CARTESIAN_POINT ( 'NONE',  ( -57.08002265617300708, 84.22855780814606419, 35.00000000000000000 ) ) ;
#16655=CARTESIAN_POINT ( 'NONE',  ( -76.88981177685832336, 91.32863676353446181, 64.92892784414958385 ) ) ;
#16666=CIRCLE ( 'NONE', #3243, 9.197489084949710403 ) ;
#16689=EDGE_CURVE ( 'NONE', #10840, #7660, #17242, .T. ) ;
#16694=ADVANCED_FACE ( 'NONE', ( #12785, #8746 ), #1711, .T. ) ;
#16708=CARTESIAN_POINT ( 'NONE',  ( -57.08002265617302839, 27.37185818390810965, 97.49999999999998579 ) ) ;
#16710=EDGE_CURVE ( 'NONE', #4505, #13449, #11981, .T. ) ;
#16712=CARTESIAN_POINT ( 'NONE',  ( -36.75995840238027768, 78.75501449464320558, 67.63319222991752611 ) ) ;
#16728=AXIS2_PLACEMENT_3D ( 'NONE', #10191, #7300, #16063 ) ;
#16732=DIRECTION ( 'NONE',  ( 1.000000000000000000, 0.000000000000000000, 0.000000000000000000 ) ) ;
#16741=CARTESIAN_POINT ( 'NONE',  ( -57.08002265617300708, 84.22855780814606419, 77.50000000000000000 ) ) ;
#16751=CARTESIAN_POINT ( 'NONE',  ( -76.98508353746098010, 91.05728076224789902, 65.61100200373311964 ) ) ;
#16765=CYLINDRICAL_SURFACE ( 'NONE', #9083, 7.500000000000000000 ) ;
#16768=SHAPE_DEFINITION_REPRESENTATION ( #4890, #14258 ) ;
#16875=ORIENTED_EDGE ( 'NONE', *, *, #5273, .F. ) ;
#16896=CARTESIAN_POINT ( 'NONE',  ( -59.22941447913690638, 106.4346967249111628, 97.49999999999998579 ) ) ;
#16951=CARTESIAN_POINT ( 'NONE',  ( -47.03642545851250389, 84.22855780814606419, -61.50000000000001421 ) ) ;
#16952=FACE_BOUND ( 'NONE', #10658, .T. ) ;
#16979=ORIENTED_EDGE ( 'NONE', *, *, #13214, .T. ) ;
#17005=ORIENTED_EDGE ( 'NONE', *, *, #17386, .T. ) ;
#17012=VERTEX_POINT ( 'NONE', #5340 ) ;
#17036=CIRCLE ( 'NONE', #3577, 42.49926016644946003 ) ;
#17051=AXIS2_PLACEMENT_3D ( 'NONE', #10188, #17651, #1953 ) ;
#17094=ORIENTED_EDGE ( 'NONE', *, *, #16710, .F. ) ;
#17147=CIRCLE ( 'NONE', #15038, 4.999999999999998224 ) ;
#17161=EDGE_CURVE ( 'NONE', #7660, #8703, #17332, .T. ) ;
#17188=LINE ( 'NONE', #6023, #8124 ) ;
#17212=DIRECTION ( 'NONE',  ( 0.000000000000000000, 0.000000000000000000, 1.000000000000000000 ) ) ;
#17214=DIRECTION ( 'NONE',  ( 1.000000000000000000, 0.000000000000000000, 0.000000000000000000 ) ) ;
#17221=DIRECTION ( 'NONE',  ( 0.000000000000000000, 0.000000000000000000, 1.000000000000000000 ) ) ;
#17229=ORIENTED_EDGE ( 'NONE', *, *, #2421, .F. ) ;
#17242=LINE ( 'NONE', #10330, #11686 ) ;
#17296=AXIS2_PLACEMENT_3D ( 'NONE', #5927, #323, #421 ) ;
#17321=ORIENTED_EDGE ( 'NONE', *, *, #14997, .T. ) ;
#17332=B_SPLINE_CURVE_WITH_KNOTS ( 'NONE', 3,
 ( #4656, #13358, #534, #1583, #7559, #14663, #15887, #13184, #17646, #13273, #10105, #11861, #17551, #3077, #15804, #2990, #4733, #7295, #4472, #8793, #1676, #5960, #4560, #7382, #13097, #11683, #358, #10278, #15983, #3172, #8883, #14576, #10453, #16148, #7464, #1758, #3339, #6047, #11774, #17471, #16060, #8969, #9064, #14751 ),
 .UNSPECIFIED., .F., .F.,
 ( 4, 2, 2, 2, 2, 2, 2, 2, 2, 2, 2, 2, 2, 2, 2, 2, 2, 2, 2, 2, 2, 4 ),
 ( 0.02364448373982099005, 0.02438320150779624967, 0.02512191927577150929, 0.02659935481172202160, 0.02807679034767253390, 0.02955422588362304273, 0.03103166141957355503, 0.03177037918754881812, 0.03250909695552409162, 0.03398653249147459698, 0.03546396802742510235, 0.03694140356337561465, 0.03768012133135086733, 0.03841883909932612695, 0.03915755686730137963, 0.03989627463527663231, 0.04137371017122716543, 0.04285114570717769855, 0.04432858124312823167, 0.04506729901110349823, 0.04580601677907876479, 0.04728345231502934648 ),
 .UNSPECIFIED. ) ;
#17334=CIRCLE ( 'NONE', #1224, 7.500000000000000000 ) ;
#17348=DIRECTION ( 'NONE',  ( -0.000000000000000000, -0.000000000000000000, 1.000000000000000000 ) ) ;
#17367=DIRECTION ( 'NONE',  ( -0.000000000000000000, -0.000000000000000000, -1.000000000000000000 ) ) ;
#17374=FACE_BOUND ( 'NONE', #12505, .T. ) ;
#17386=EDGE_CURVE ( 'NONE', #13818, #18509, #17188, .T. ) ;
#17409=TOROIDAL_SURFACE ( 'NONE', #13537, 47.49926016644912607, 5.000000000000000000 ) ;
#17469=CARTESIAN_POINT ( 'NONE',  ( -46.03642545851250389, 84.22855780814606419, 68.73600986863397111 ) ) ;
#17471=CARTESIAN_POINT ( 'NONE',  ( -36.12567045178374059, 86.17903909013999453, 55.25386615338222640 ) ) ;
#17510=ORIENTED_EDGE ( 'NONE', *, *, #15805, .T. ) ;
#17519=ORIENTED_EDGE ( 'NONE', *, *, #803, .T. ) ;
#17520=CYLINDRICAL_SURFACE ( 'NONE', #11605, 7.500000000000000000 ) ;
#17539=DIRECTION ( 'NONE',  ( 0.000000000000000000, 0.000000000000000000, -1.000000000000000000 ) ) ;
#17551=CARTESIAN_POINT ( 'NONE',  ( -36.89658380969908791, 90.19024662095814904, 67.07644706209384822 ) ) ;
#17555=DIRECTION ( 'NONE',  ( 1.000000000000000000, 0.000000000000000000, 0.000000000000000000 ) ) ;
#17565=CARTESIAN_POINT ( 'NONE',  ( -77.98461495213935279, 81.80210967128928701, 69.60095798084290664 ) ) ;
#17574=DIRECTION ( 'NONE',  ( 0.000000000000000000, 0.000000000000000000, 1.000000000000000000 ) ) ;
#17579=ORIENTED_EDGE ( 'NONE', *, *, #9516, .T. ) ;
#17594=CARTESIAN_POINT ( 'NONE',  ( -77.35352728739614747, 89.88064937530401721, 57.54580211461716743 ) ) ;
#17596=FACE_OUTER_BOUND ( 'NONE', #10302, .T. ) ;
#17599=CARTESIAN_POINT ( 'NONE',  ( -57.08002265617300708, 84.22855780814606419, -61.50000000000001421 ) ) ;
#17639=DIRECTION ( 'NONE',  ( 1.000000000000000000, 0.000000000000000000, 0.000000000000000000 ) ) ;
#17646=CARTESIAN_POINT ( 'NONE',  ( -36.37372457221012922, 88.00379445693184266, 68.99882519264671998 ) ) ;
#17651=DIRECTION ( 'NONE',  ( 0.000000000000000000, 0.000000000000000000, 1.000000000000000000 ) ) ;
#17670=CARTESIAN_POINT ( 'NONE',  ( -7.840676406241780860, 112.6569076202650308, 97.49999999999998579 ) ) ;
#17671=DIRECTION ( 'NONE',  ( 1.000000000000000000, 0.000000000000000000, 0.000000000000000000 ) ) ;
#17690=CARTESIAN_POINT ( 'NONE',  ( -57.08002265617300708, 84.22855780814606419, -62.50000000000000000 ) ) ;
#17691=ORIENTED_EDGE ( 'NONE', *, *, #12712, .T. ) ;
#17733=EDGE_CURVE ( 'NONE', #5564, #17891, #6643, .T. ) ;
#17754=VECTOR ( 'NONE', #7217, 1000.000000000000000 ) ;
#17785=ADVANCED_FACE ( 'NONE', ( #6975 ), #1097, .T. ) ;
#17795=CARTESIAN_POINT ( 'NONE',  ( -78.10200533711912385, 85.21341043856777731, 55.06082720658116614 ) ) ;
#17811=ORIENTED_EDGE ( 'NONE', *, *, #9237, .F. ) ;
#17821=EDGE_LOOP ( 'NONE', ( #11574, #11540, #10812, #1380, #13425, #219, #3957, #13986 ) ) ;
#17843=DIRECTION ( 'NONE',  ( -1.000000000000000000, 0.000000000000000000, 0.000000000000000000 ) ) ;
#17844=CARTESIAN_POINT ( 'NONE',  ( -37.06518108615770046, 77.72307496574234165, 58.73557318418679785 ) ) ;
#17856=CARTESIAN_POINT ( 'NONE',  ( -57.08002265617301418, 106.1506877598988154, 92.50000000000000000 ) ) ;
#17862=DIRECTION ( 'NONE',  ( -0.000000000000000000, -0.000000000000000000, -1.000000000000000000 ) ) ;
#17870=DIRECTION ( 'NONE',  ( 0.000000000000000000, 0.000000000000000000, 1.000000000000000000 ) ) ;
#17878=CARTESIAN_POINT ( 'NONE',  ( -76.74178926456770000, 91.72841893195355567, 62.99632217189364525 ) ) ;
#17891=VERTEX_POINT ( 'NONE', #15068 ) ;
#17909=DIRECTION ( 'NONE',  ( 1.000000000000000000, 0.000000000000000000, 0.000000000000000000 ) ) ;
#17930=DIRECTION ( 'NONE',  ( -1.000000000000000000, 0.000000000000000000, 0.000000000000000000 ) ) ;
#17932=CARTESIAN_POINT ( 'NONE',  ( -36.80564135947743409, 78.57985073358729267, 57.54245165641173543 ) ) ;
#17936=CARTESIAN_POINT ( 'NONE',  ( -76.06514409945376087, 73.26749283226919829, 102.5000000000000000 ) ) ;
#17956=CARTESIAN_POINT ( 'NONE',  ( -78.12361985383350316, 84.22855780814606419, 55.00000000000001421 ) ) ;
#17960=EDGE_CURVE ( 'NONE', #10840, #2786, #12028, .T. ) ;
#17963=CIRCLE ( 'NONE', #11123, 10.04359719766049430 ) ;
#17964=ORIENTED_EDGE ( 'NONE', *, *, #3310, .F. ) ;
#17991=LINE ( 'NONE', #8364, #4870 ) ;
#18005=EDGE_LOOP ( 'NONE', ( #10935, #11569, #7973, #16479 ) ) ;
#18007=VECTOR ( 'NONE', #16098, 1000.000000000000000 ) ;
#18019=CARTESIAN_POINT ( 'NONE',  ( -77.01829067351829394, 77.49513323845336288, 59.15998809532618452 ) ) ;
#18035=PLANE ( 'NONE',  #7486 ) ;
#18049=DIRECTION ( 'NONE',  ( 0.000000000000000000, 0.000000000000000000, 1.000000000000000000 ) ) ;
#18063=CIRCLE ( 'NONE', #3735, 2.168074330099287295 ) ;
#18082=CARTESIAN_POINT ( 'NONE',  ( -78.12361985383350316, 84.72841810161551734, 70.00000000000001421 ) ) ;
#18085=CIRCLE ( 'NONE', #4045, 7.168074330098860969 ) ;
#18137=CYLINDRICAL_SURFACE ( 'NONE', #9275, 11.04359719766049430 ) ;
#18169=ORIENTED_EDGE ( 'NONE', *, *, #12610, .T. ) ;
#18172=CARTESIAN_POINT ( 'NONE',  ( -78.03437486056226646, 86.17903909013998032, 69.74613384661780913 ) ) ;
#18228=FACE_OUTER_BOUND ( 'NONE', #5367, .T. ) ;
#18232=CIRCLE ( 'NONE', #13148, 7.500000000000000000 ) ;
#18233=ORIENTED_EDGE ( 'NONE', *, *, #9237, .T. ) ;
#18239=ORIENTED_EDGE ( 'NONE', *, *, #6156, .F. ) ;
#18254=CIRCLE ( 'NONE', #16440, 11.04359719766050141 ) ;
#18257=VECTOR ( 'NONE', #9995, 1000.000000000000000 ) ;
#18283=ORIENTED_EDGE ( 'NONE', *, *, #15403, .T. ) ;
#18332=FACE_OUTER_BOUND ( 'NONE', #7364, .T. ) ;
#18365=DIRECTION ( 'NONE',  ( -0.000000000000000000, -0.000000000000000000, -1.000000000000000000 ) ) ;
#18368=PLANE ( 'NONE',  #647 ) ;
#18398=FACE_OUTER_BOUND ( 'NONE', #872, .T. ) ;
#18399=DIRECTION ( 'NONE',  ( -1.000000000000000000, 0.000000000000000000, 0.000000000000000000 ) ) ;
#18405=EDGE_LOOP ( 'NONE', ( #6142, #18283, #9647, #5396 ) ) ;
#18418=LINE ( 'NONE', #2963, #11391 ) ;
#18429=ORIENTED_EDGE ( 'NONE', *, *, #16245, .F. ) ;
#18469=ORIENTED_EDGE ( 'NONE', *, *, #16245, .T. ) ;
#18479=DIRECTION ( 'NONE',  ( -1.000000000000000000, 0.000000000000000000, 0.000000000000000000 ) ) ;
#18493=CARTESIAN_POINT ( 'NONE',  ( -80.43148536604020649, 78.95224028009165806, 97.49999999999998579 ) ) ;
#18495=DIRECTION ( 'NONE',  ( 1.000000000000000000, 0.000000000000000000, 0.000000000000000000 ) ) ;
#18509=VERTEX_POINT ( 'NONE', #259 ) ;
#18567=COLOUR_RGB('Off White',0.89,0.88,0.83);
#18568=FILL_AREA_STYLE_COLOUR('',#18567);
#18569=FILL_AREA_STYLE('',(#18568));
#18570=SURFACE_STYLE_FILL_AREA(#18569);
#18571=SURFACE_SIDE_STYLE('',(#18570));
#18572=SURFACE_STYLE_USAGE(.BOTH.,#18571);
#18573=PRESENTATION_STYLE_ASSIGNMENT((#18572));
ENDSEC;
END-ISO-10303-21;
